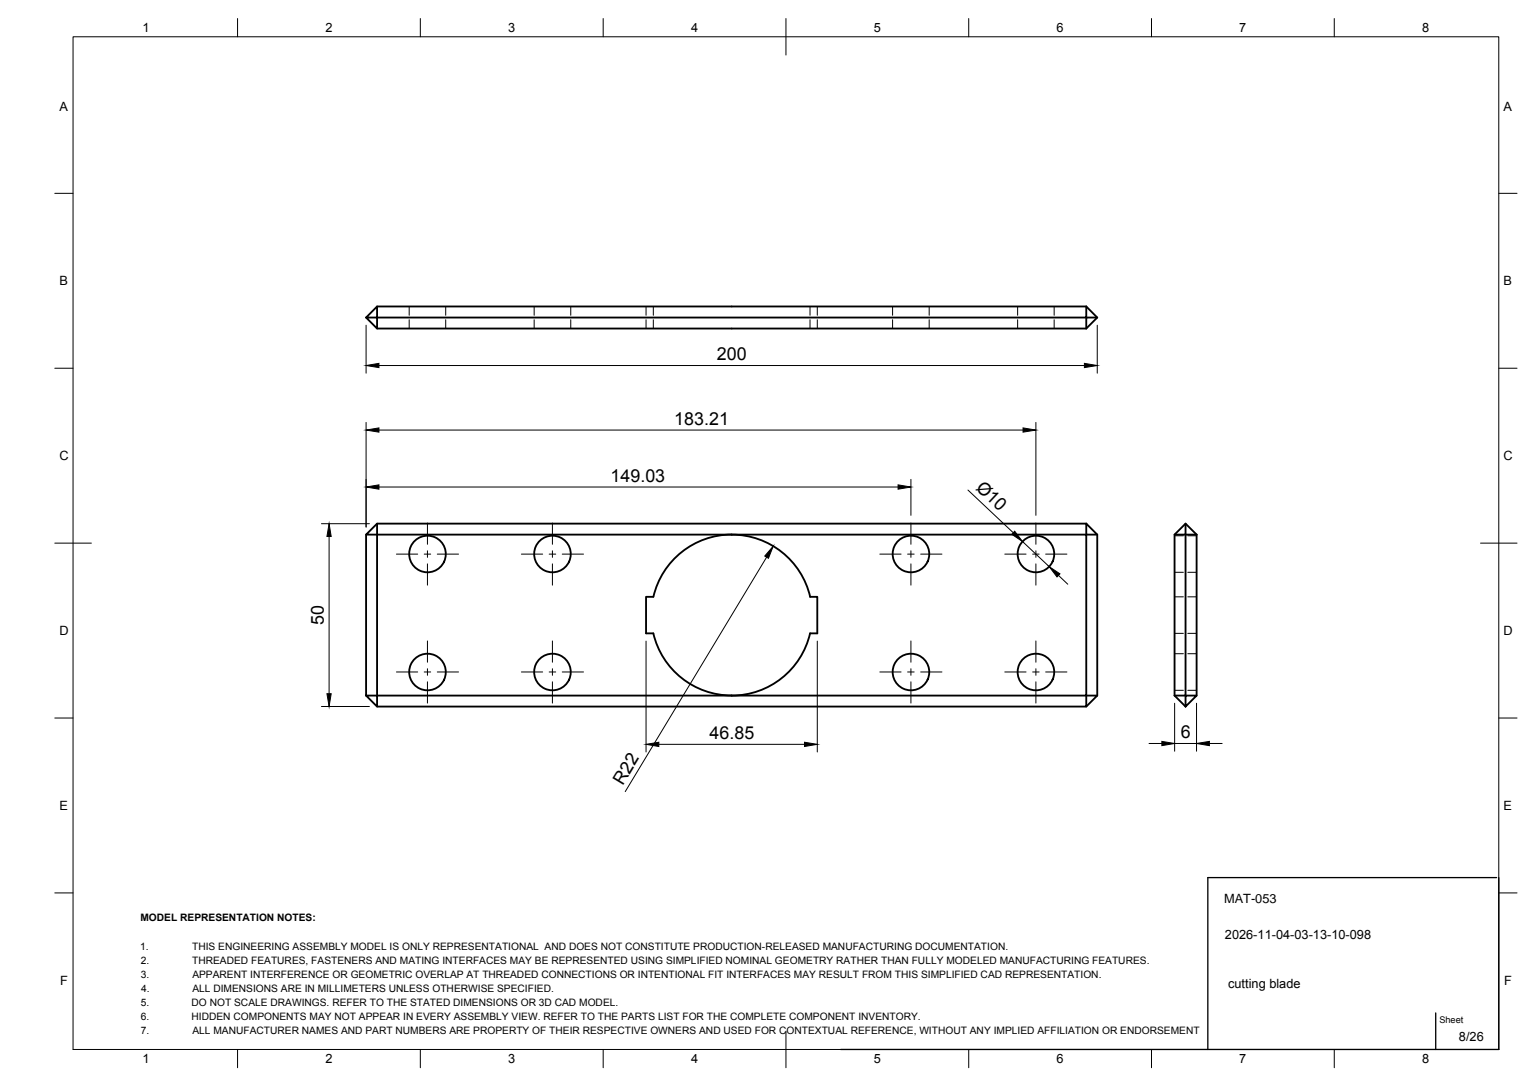
ISO-10303-21;
HEADER;
FILE_DESCRIPTION (('STEP AP214'),
    '1' );
FILE_NAME ('cutting blade.step',
    '2026-10-10T03:43:58',
    ( '' ),
    ( '' ),
    'SwSTEP 2.0',
    'SolidWorks 2026',
    '' );
FILE_SCHEMA (( 'AUTOMOTIVE_DESIGN' ));
ENDSEC;

DATA;
#169=CARTESIAN_POINT ( 'NONE',  ( 123.4242852856285566, 6.000000000000000000, 0.000000000000000000 ) ) ;
#175=PLANE ( 'NONE',  #51290 ) ;
#357=AXIS2_PLACEMENT_3D ( 'NONE', #51385, #66883, #65837 ) ;
#396=ORIENTED_EDGE ( 'NONE', *, *, #36645, .T. ) ;
#421=VECTOR ( 'NONE', #35144, 1000.000000000000000 ) ;
#435=APPLICATION_CONTEXT ( 'automotive_design' ) ;
#494=FACE_OUTER_BOUND ( 'NONE', #26933, .T. ) ;
#533=LINE ( 'NONE', #52947, #16766 ) ;
#715=CARTESIAN_POINT ( 'NONE',  ( 200.0000000000000000, 2.999999999999969802, -46.99999999999997158 ) ) ;
#779=CARTESIAN_POINT ( 'NONE',  ( 196.9999999999999716, 1.500000000000015321, -1.500000000000015321 ) ) ;
#839=DIRECTION ( 'NONE',  ( 0.7071067811865475727, 0.000000000000000000, -0.7071067811865475727 ) ) ;
#878=LINE ( 'NONE', #59590, #42830 ) ;
#897=CARTESIAN_POINT ( 'NONE',  ( 0.000000000000000000, 6.000000000000000000, -46.99999999999997158 ) ) ;
#978=DIRECTION ( 'NONE',  ( -0.000000000000000000, -1.000000000000000000, -0.000000000000000000 ) ) ;
#1008=LINE ( 'NONE', #43202, #21889 ) ;
#1056=CYLINDRICAL_SURFACE ( 'NONE', #3184, 5.000000000000018652 ) ;
#1109=CIRCLE ( 'NONE', #48227, 21.99999999999998579 ) ;
#1145=DIRECTION ( 'NONE',  ( -0.000000000000000000, -0.7071067811865474617, 0.7071067811865474617 ) ) ;
#1186=FACE_BOUND ( 'NONE', #2757, .T. ) ;
#1201=DIRECTION ( 'NONE',  ( -0.5773502691896255090, -0.5773502691896258421, 0.5773502691896258421 ) ) ;
#1207=ADVANCED_FACE ( 'NONE', ( #57854, #55337, #28257, #1186, #27560 ), #44439, .F. ) ;
#1231=LINE ( 'NONE', #29025, #57253 ) ;
#1239=DIRECTION ( 'NONE',  ( 0.7071067811865474617, -0.7071067811865474617, -0.000000000000000000 ) ) ;
#1254=VERTEX_POINT ( 'NONE', #27212 ) ;
#1260=EDGE_CURVE ( 'NONE', #42425, #65549, #28621, .T. ) ;
#1315=PLANE ( 'NONE',  #1532 ) ;
#1431=DIRECTION ( 'NONE',  ( 0.000000000000000000, 1.000000000000000000, 0.000000000000000000 ) ) ;
#1515=DIRECTION ( 'NONE',  ( 0.000000000000000000, 1.000000000000000000, -0.000000000000000000 ) ) ;
#1532=AXIS2_PLACEMENT_3D ( 'NONE', #12569, #6939, #17848 ) ;
#1616=ORIENTED_EDGE ( 'NONE', *, *, #7716, .T. ) ;
#1626=CARTESIAN_POINT ( 'NONE',  ( 16.78635691501517613, 6.000000000000000000, -4.435653166495499455 ) ) ;
#1709=CARTESIAN_POINT ( 'NONE',  ( 200.0000000000000000, 0.000000000000000000, -46.99999999999997158 ) ) ;
#1740=VECTOR ( 'NONE', #65545, 1000.000000000000000 ) ;
#1772=ORIENTED_EDGE ( 'NONE', *, *, #31156, .T. ) ;
#1902=DIRECTION ( 'NONE',  ( 0.000000000000000000, 0.000000000000000000, -1.000000000000000000 ) ) ;
#1942=CARTESIAN_POINT ( 'NONE',  ( 50.97490815085634352, 6.000000000000000000, -46.68900338898716029 ) ) ;
#1982=AXIS2_PLACEMENT_3D ( 'NONE', #37710, #69378, #69021 ) ;
#2065=CARTESIAN_POINT ( 'NONE',  ( 78.57571471437144339, 0.000000000000000000, -30.00000000000000355 ) ) ;
#2169=DIRECTION ( 'NONE',  ( -0.7071067811865474617, -0.000000000000000000, -0.7071067811865474617 ) ) ;
#2253=DIRECTION ( 'NONE',  ( 0.000000000000000000, 0.000000000000000000, -1.000000000000000000 ) ) ;
#2282=CARTESIAN_POINT ( 'NONE',  ( 183.2136430849847955, 6.000000000000000000, -41.68900338898720292 ) ) ;
#2313=CIRCLE ( 'NONE', #61839, 21.99999999999998579 ) ;
#2414=DIRECTION ( 'NONE',  ( 0.000000000000000000, 1.000000000000000000, -0.000000000000000000 ) ) ;
#2441=PLANE ( 'NONE',  #40587 ) ;
#2448=AXIS2_PLACEMENT_3D ( 'NONE', #61221, #56632, #34153 ) ;
#2451=DIRECTION ( 'NONE',  ( -0.000000000000000000, -1.000000000000000000, -0.000000000000000000 ) ) ;
#2481=EDGE_CURVE ( 'NONE', #65549, #11659, #47136, .T. ) ;
#2566=ORIENTED_EDGE ( 'NONE', *, *, #63693, .F. ) ;
#2616=DIRECTION ( 'NONE',  ( -0.7071067811865474617, 0.7071067811865474617, -0.000000000000000000 ) ) ;
#2621=ORIENTED_EDGE ( 'NONE', *, *, #25957, .T. ) ;
#2671=DIRECTION ( 'NONE',  ( -0.000000000000000000, -1.000000000000000000, -0.000000000000000000 ) ) ;
#2707=FACE_OUTER_BOUND ( 'NONE', #53949, .T. ) ;
#2757=EDGE_LOOP ( 'NONE', ( #15220, #28245 ) ) ;
#2839=CARTESIAN_POINT ( 'NONE',  ( 183.2136430849848239, 0.000000000000000000, -14.43565316649556074 ) ) ;
#3063=EDGE_LOOP ( 'NONE', ( #65576, #48668, #15693, #29611 ) ) ;
#3184=AXIS2_PLACEMENT_3D ( 'NONE', #43604, #65785, #22507 ) ;
#3357=ORIENTED_EDGE ( 'NONE', *, *, #27947, .T. ) ;
#3410=VECTOR ( 'NONE', #2671, 1000.000000000000000 ) ;
#3435=AXIS2_PLACEMENT_3D ( 'NONE', #57257, #35805, #24215 ) ;
#3493=EDGE_CURVE ( 'NONE', #67476, #41408, #39123, .T. ) ;
#3530=ORIENTED_EDGE ( 'NONE', *, *, #45276, .F. ) ;
#3676=LINE ( 'NONE', #56449, #63447 ) ;
#3686=DIRECTION ( 'NONE',  ( 0.000000000000000000, 0.000000000000000000, -1.000000000000000000 ) ) ;
#3694=ORIENTED_EDGE ( 'NONE', *, *, #20467, .T. ) ;
#3705=EDGE_LOOP ( 'NONE', ( #55339, #15386, #56019, #65378, #27658 ) ) ;
#3834=EDGE_CURVE ( 'NONE', #64271, #1254, #23024, .T. ) ;
#3913=VERTEX_POINT ( 'NONE', #61691 ) ;
#3955=DIRECTION ( 'NONE',  ( -0.000000000000000000, -1.000000000000000000, -0.000000000000000000 ) ) ;
#4029=CARTESIAN_POINT ( 'NONE',  ( 200.0000000000000000, 3.000000000000030198, -3.000000000000030198 ) ) ;
#4101=EDGE_LOOP ( 'NONE', ( #34045, #40743 ) ) ;
#4168=ORIENTED_EDGE ( 'NONE', *, *, #18126, .T. ) ;
#4278=ORIENTED_EDGE ( 'NONE', *, *, #64901, .F. ) ;
#4281=ORIENTED_EDGE ( 'NONE', *, *, #27062, .T. ) ;
#4315=CARTESIAN_POINT ( 'NONE',  ( 16.78635691501517613, 0.000000000000000000, -4.435653166495499455 ) ) ;
#4420=DIRECTION ( 'NONE',  ( 1.000000000000000000, -0.000000000000000000, -0.000000000000000000 ) ) ;
#4432=EDGE_CURVE ( 'NONE', #53754, #46832, #13689, .T. ) ;
#4537=DIRECTION ( 'NONE',  ( 0.000000000000000000, 1.000000000000000000, -0.000000000000000000 ) ) ;
#4544=CYLINDRICAL_SURFACE ( 'NONE', #15389, 5.000000000000000888 ) ;
#4601=ADVANCED_FACE ( 'NONE', ( #54409 ), #1315, .F. ) ;
#4627=AXIS2_PLACEMENT_3D ( 'NONE', #8850, #67257, #25026 ) ;
#4646=DIRECTION ( 'NONE',  ( 0.000000000000000000, 0.000000000000000000, 1.000000000000000000 ) ) ;
#4723=FACE_OUTER_BOUND ( 'NONE', #69286, .T. ) ;
#4726=ORIENTED_EDGE ( 'NONE', *, *, #60338, .T. ) ;
#4768=DIRECTION ( 'NONE',  ( 1.000000000000000000, 0.000000000000000000, 1.734723475976805517E-15 ) ) ;
#4785=EDGE_LOOP ( 'NONE', ( #23234, #53980 ) ) ;
#4794=DIRECTION ( 'NONE',  ( 0.000000000000000000, 0.000000000000000000, -1.000000000000000000 ) ) ;
#4937=CARTESIAN_POINT ( 'NONE',  ( 5.204170427930454100E-14, 6.000000000000000000, -30.00000000000021316 ) ) ;
#4941=AXIS2_PLACEMENT_3D ( 'NONE', #7124, #6773, #39149 ) ;
#4955=FACE_OUTER_BOUND ( 'NONE', #64021, .T. ) ;
#5076=EDGE_CURVE ( 'NONE', #50492, #67476, #66494, .T. ) ;
#5099=CARTESIAN_POINT ( 'NONE',  ( 149.0250918491436778, 0.000000000000000000, -4.435653166495538535 ) ) ;
#5123=AXIS2_PLACEMENT_3D ( 'NONE', #5757, #63827, #58199 ) ;
#5128=DIRECTION ( 'NONE',  ( -1.000000000000000000, 0.000000000000000000, 0.000000000000000000 ) ) ;
#5242=ORIENTED_EDGE ( 'NONE', *, *, #14158, .F. ) ;
#5316=LINE ( 'NONE', #10238, #50013 ) ;
#5338=CARTESIAN_POINT ( 'NONE',  ( 123.4242852856285566, 10.00000000000000000, -30.00000000000000000 ) ) ;
#5431=FACE_OUTER_BOUND ( 'NONE', #59546, .T. ) ;
#5461=EDGE_CURVE ( 'NONE', #17220, #64271, #10143, .T. ) ;
#5496=CARTESIAN_POINT ( 'NONE',  ( 76.57571471437145760, 0.000000000000000000, -30.00000000000000000 ) ) ;
#5497=FACE_BOUND ( 'NONE', #67109, .T. ) ;
#5558=ORIENTED_EDGE ( 'NONE', *, *, #20467, .F. ) ;
#5597=CIRCLE ( 'NONE', #40459, 5.000000000000018652 ) ;
#5637=ORIENTED_EDGE ( 'NONE', *, *, #14756, .T. ) ;
#5640=VERTEX_POINT ( 'NONE', #9729 ) ;
#5740=FACE_OUTER_BOUND ( 'NONE', #30395, .T. ) ;
#5757=CARTESIAN_POINT ( 'NONE',  ( 183.2136430849848239, 6.000000000000000000, -9.435653166495541200 ) ) ;
#5788=CIRCLE ( 'NONE', #2448, 4.999999999999990230 ) ;
#5944=VERTEX_POINT ( 'NONE', #17776 ) ;
#5971=VECTOR ( 'NONE', #26457, 1000.000000000000000 ) ;
#6015=AXIS2_PLACEMENT_3D ( 'NONE', #62685, #18728, #40188 ) ;
#6027=CYLINDRICAL_SURFACE ( 'NONE', #52139, 4.999999999999990230 ) ;
#6089=ORIENTED_EDGE ( 'NONE', *, *, #12217, .F. ) ;
#6097=DIRECTION ( 'NONE',  ( -0.000000000000000000, -0.7071067811865474617, -0.7071067811865474617 ) ) ;
#6148=VERTEX_POINT ( 'NONE', #9291 ) ;
#6166=EDGE_CURVE ( 'NONE', #44138, #3913, #52873, .T. ) ;
#6181=( GEOMETRIC_REPRESENTATION_CONTEXT ( 3 ) GLOBAL_UNCERTAINTY_ASSIGNED_CONTEXT ( ( #62024 ) ) GLOBAL_UNIT_ASSIGNED_CONTEXT ( ( #51907, #14959, #58221 ) ) REPRESENTATION_CONTEXT ( 'NONE', 'WORKASPACE' ) );
#6323=EDGE_CURVE ( 'NONE', #30445, #36476, #50644, .T. ) ;
#6355=CARTESIAN_POINT ( 'NONE',  ( 3.000000000000028866, 2.999999999999969802, 0.000000000000000000 ) ) ;
#6420=CARTESIAN_POINT ( 'NONE',  ( 196.9999999999999716, 2.999999999999969802, 0.000000000000000000 ) ) ;
#6461=EDGE_CURVE ( 'NONE', #60670, #23191, #10490, .T. ) ;
#6509=ORIENTED_EDGE ( 'NONE', *, *, #37316, .F. ) ;
#6538=ORIENTED_EDGE ( 'NONE', *, *, #17367, .T. ) ;
#6617=CARTESIAN_POINT ( 'NONE',  ( 50.97490815085634352, 6.000000000000000000, -41.68900338898716740 ) ) ;
#6648=EDGE_CURVE ( 'NONE', #36476, #52936, #41005, .T. ) ;
#6690=VERTEX_POINT ( 'NONE', #8674 ) ;
#6773=DIRECTION ( 'NONE',  ( -1.000000000000000000, 0.000000000000000000, 0.000000000000000000 ) ) ;
#6818=EDGE_LOOP ( 'NONE', ( #40697, #28804, #34762, #10078 ) ) ;
#6835=LINE ( 'NONE', #32189, #53156 ) ;
#6843=CIRCLE ( 'NONE', #67521, 4.999999999999990230 ) ;
#6939=DIRECTION ( 'NONE',  ( -1.734723475976805517E-15, 0.000000000000000000, -1.000000000000000000 ) ) ;
#6948=AXIS2_PLACEMENT_3D ( 'NONE', #19833, #41289, #36353 ) ;
#6972=CARTESIAN_POINT ( 'NONE',  ( 0.000000000000000000, 6.000000000000000000, -46.99999999999997158 ) ) ;
#6986=EDGE_CURVE ( 'NONE', #6690, #44138, #3676, .T. ) ;
#7064=LINE ( 'NONE', #33103, #61226 ) ;
#7089=VERTEX_POINT ( 'NONE', #32140 ) ;
#7104=DIRECTION ( 'NONE',  ( 0.000000000000000000, 0.000000000000000000, 1.000000000000000000 ) ) ;
#7108=CIRCLE ( 'NONE', #14983, 5.000000000000018652 ) ;
#7124=CARTESIAN_POINT ( 'NONE',  ( 123.4242852856285566, 10.00000000000000000, -20.00000000000000000 ) ) ;
#7145=ORIENTED_EDGE ( 'NONE', *, *, #29514, .T. ) ;
#7165=EDGE_CURVE ( 'NONE', #45847, #62711, #39167, .T. ) ;
#7169=VECTOR ( 'NONE', #47823, 1000.000000000000114 ) ;
#7198=CARTESIAN_POINT ( 'NONE',  ( 198.4999999999999716, 4.499999999999984901, -3.000000000000030198 ) ) ;
#7220=VECTOR ( 'NONE', #55627, 1000.000000000000114 ) ;
#7324=EDGE_CURVE ( 'NONE', #42425, #30796, #49253, .T. ) ;
#7466=CARTESIAN_POINT ( 'NONE',  ( 149.0250918491436494, 6.000000000000000000, -36.68900338898720292 ) ) ;
#7473=CIRCLE ( 'NONE', #20911, 4.999999999999990230 ) ;
#7553=LINE ( 'NONE', #44477, #68985 ) ;
#7574=ORIENTED_EDGE ( 'NONE', *, *, #3834, .F. ) ;
#7587=CARTESIAN_POINT ( 'NONE',  ( 196.9999999999999716, 4.499999999999984901, -48.49999999999998579 ) ) ;
#7647=DIRECTION ( 'NONE',  ( 0.000000000000000000, 0.000000000000000000, -1.000000000000000000 ) ) ;
#7685=ORIENTED_EDGE ( 'NONE', *, *, #32000, .T. ) ;
#7701=DIRECTION ( 'NONE',  ( 0.000000000000000000, 1.000000000000000000, 0.000000000000000000 ) ) ;
#7716=EDGE_CURVE ( 'NONE', #10774, #9838, #42015, .T. ) ;
#7755=VECTOR ( 'NONE', #58395, 1000.000000000000000 ) ;
#7779=EDGE_CURVE ( 'NONE', #44138, #63882, #58869, .T. ) ;
#8093=EDGE_CURVE ( 'NONE', #30336, #59608, #10600, .T. ) ;
#8143=ORIENTED_EDGE ( 'NONE', *, *, #37114, .F. ) ;
#8183=CARTESIAN_POINT ( 'NONE',  ( 3.000000000000028866, 3.000000000000030198, 0.000000000000000000 ) ) ;
#8253=( GEOMETRIC_REPRESENTATION_CONTEXT ( 3 ) GLOBAL_UNCERTAINTY_ASSIGNED_CONTEXT ( ( #56404 ) ) GLOBAL_UNIT_ASSIGNED_CONTEXT ( ( #66641, #61689, #39207 ) ) REPRESENTATION_CONTEXT ( 'NONE', 'WORKASPACE' ) );
#8319=DIRECTION ( 'NONE',  ( 1.000000000000000000, 0.000000000000000000, 0.000000000000000000 ) ) ;
#8373=DIRECTION ( 'NONE',  ( 0.000000000000000000, 0.000000000000000000, -1.000000000000000000 ) ) ;
#8472=FACE_OUTER_BOUND ( 'NONE', #38130, .T. ) ;
#8514=VECTOR ( 'NONE', #4420, 1000.000000000000000 ) ;
#8518=AXIS2_PLACEMENT_3D ( 'NONE', #27196, #47274, #47958 ) ;
#8530=EDGE_CURVE ( 'NONE', #53590, #18148, #7473, .T. ) ;
#8544=PLANE ( 'NONE',  #22300 ) ;
#8547=LINE ( 'NONE', #58106, #60205 ) ;
#8625=ORIENTED_EDGE ( 'NONE', *, *, #32000, .F. ) ;
#8629=DIRECTION ( 'NONE',  ( 0.000000000000000000, -0.7071067811865474617, 0.7071067811865474617 ) ) ;
#8637=DIRECTION ( 'NONE',  ( 0.000000000000000000, -1.000000000000000000, 0.000000000000000000 ) ) ;
#8674=CARTESIAN_POINT ( 'NONE',  ( 3.000000000000028866, 6.000000000000000000, -3.000000000000030198 ) ) ;
#8754=DIRECTION ( 'NONE',  ( -0.000000000000000000, -1.000000000000000000, -0.000000000000000000 ) ) ;
#8806=DIRECTION ( 'NONE',  ( 0.000000000000000000, 0.000000000000000000, -1.000000000000000000 ) ) ;
#8824=DIRECTION ( 'NONE',  ( 0.000000000000000000, 1.000000000000000000, 0.000000000000000000 ) ) ;
#8850=CARTESIAN_POINT ( 'NONE',  ( -2.775557561562891351E-14, 3.000000000000030198, -50.00000000000000000 ) ) ;
#8855=ORIENTED_EDGE ( 'NONE', *, *, #12862, .F. ) ;
#8968=VERTEX_POINT ( 'NONE', #60893 ) ;
#9045=EDGE_LOOP ( 'NONE', ( #5242, #53942, #39507, #50271 ) ) ;
#9066=CARTESIAN_POINT ( 'NONE',  ( 121.4242852856285566, 6.000000000000000000, -20.00000000000000000 ) ) ;
#9085=DIRECTION ( 'NONE',  ( 0.000000000000000000, 0.000000000000000000, -1.000000000000000000 ) ) ;
#9124=AXIS2_PLACEMENT_3D ( 'NONE', #12076, #1515, #28240 ) ;
#9125=AXIS2_PLACEMENT_3D ( 'NONE', #27577, #1201, #49369 ) ;
#9291=CARTESIAN_POINT ( 'NONE',  ( 78.57571471437145760, 0.000000000000000000, -20.00000000000000000 ) ) ;
#9319=DIRECTION ( 'NONE',  ( -0.5773502691896258421, -0.5773502691896258421, -0.5773502691896258421 ) ) ;
#9380=ADVANCED_FACE ( 'NONE', ( #36213 ), #31622, .F. ) ;
#9400=ORIENTED_EDGE ( 'NONE', *, *, #44188, .T. ) ;
#9421=ORIENTED_EDGE ( 'NONE', *, *, #64314, .T. ) ;
#9457=ADVANCED_FACE ( 'NONE', ( #20369 ), #4544, .F. ) ;
#9513=CIRCLE ( 'NONE', #54419, 21.99999999999998579 ) ;
#9591=EDGE_LOOP ( 'NONE', ( #62598, #61913, #37505, #11408, #50798, #48930, #15590, #30937 ) ) ;
#9674=VECTOR ( 'NONE', #6097, 1000.000000000000114 ) ;
#9729=CARTESIAN_POINT ( 'NONE',  ( -2.609024107869115977E-14, 3.000000000000030198, -46.99999999999997158 ) ) ;
#9838=VERTEX_POINT ( 'NONE', #32576 ) ;
#9897=CYLINDRICAL_SURFACE ( 'NONE', #31651, 21.99999999999998579 ) ;
#10012=DIRECTION ( 'NONE',  ( 1.000000000000000000, 0.000000000000000000, 0.000000000000000000 ) ) ;
#10024=PLANE ( 'NONE',  #29251 ) ;
#10078=ORIENTED_EDGE ( 'NONE', *, *, #33445, .F. ) ;
#10104=DIRECTION ( 'NONE',  ( 0.000000000000000000, 0.000000000000000000, -1.000000000000000000 ) ) ;
#10143=LINE ( 'NONE', #59362, #36435 ) ;
#10216=DIRECTION ( 'NONE',  ( -0.7071067811865474617, 0.7071067811865474617, 0.000000000000000000 ) ) ;
#10224=CARTESIAN_POINT ( 'NONE',  ( 99.99999999999997158, 6.000000000000000000, -25.00000000000000000 ) ) ;
#10238=CARTESIAN_POINT ( 'NONE',  ( 16.78635691501517613, 6.000000000000000000, -36.68900338898716740 ) ) ;
#10314=ORIENTED_EDGE ( 'NONE', *, *, #42088, .F. ) ;
#10378=PRODUCT_CONTEXT ( 'NONE', #41742, 'mechanical' ) ;
#10389=EDGE_CURVE ( 'NONE', #41408, #31811, #31037, .T. ) ;
#10396=CIRCLE ( 'NONE', #36269, 4.999999999999996447 ) ;
#10399=PLANE ( 'NONE',  #11397 ) ;
#10422=PLANE ( 'NONE',  #35855 ) ;
#10452=ORIENTED_EDGE ( 'NONE', *, *, #18428, .F. ) ;
#10477=LINE ( 'NONE', #47764, #48342 ) ;
#10488=VERTEX_POINT ( 'NONE', #26095 ) ;
#10490=LINE ( 'NONE', #47427, #26395 ) ;
#10542=ADVANCED_FACE ( 'NONE', ( #51456 ), #40889, .F. ) ;
#10543=EDGE_LOOP ( 'NONE', ( #41686, #46294, #63996, #41184, #25059 ) ) ;
#10600=LINE ( 'NONE', #5338, #11868 ) ;
#10607=DIRECTION ( 'NONE',  ( 0.7071067811865475727, -0.7071067811865475727, 0.000000000000000000 ) ) ;
#10749=CIRCLE ( 'NONE', #52337, 4.999999999999997335 ) ;
#10774=VERTEX_POINT ( 'NONE', #9066 ) ;
#10905=EDGE_LOOP ( 'NONE', ( #65462, #4726, #57157, #8855 ) ) ;
#10968=CARTESIAN_POINT ( 'NONE',  ( 196.9999999999999716, 1.500000000000015321, -48.49999999999998579 ) ) ;
#11042=DIRECTION ( 'NONE',  ( -0.000000000000000000, -1.000000000000000000, -0.000000000000000000 ) ) ;
#11068=ORIENTED_EDGE ( 'NONE', *, *, #54016, .F. ) ;
#11085=PLANE ( 'NONE',  #16711 ) ;
#11100=CARTESIAN_POINT ( 'NONE',  ( 50.97490815085634352, 6.000000000000000000, -9.435653166495500344 ) ) ;
#11157=VECTOR ( 'NONE', #55500, 1000.000000000000000 ) ;
#11216=DIRECTION ( 'NONE',  ( 0.000000000000000000, -0.7071067811865475727, 0.7071067811865475727 ) ) ;
#11232=ORIENTED_EDGE ( 'NONE', *, *, #23537, .F. ) ;
#11246=DIRECTION ( 'NONE',  ( 0.000000000000000000, 1.000000000000000000, 0.000000000000000000 ) ) ;
#11328=ADVANCED_FACE ( 'NONE', ( #494 ), #64865, .F. ) ;
#11329=ORIENTED_EDGE ( 'NONE', *, *, #32716, .T. ) ;
#11389=CARTESIAN_POINT ( 'NONE',  ( 0.000000000000000000, 6.000000000000000000, -3.000000000000030198 ) ) ;
#11397=AXIS2_PLACEMENT_3D ( 'NONE', #37835, #5128, #64569 ) ;
#11408=ORIENTED_EDGE ( 'NONE', *, *, #24486, .F. ) ;
#11474=CARTESIAN_POINT ( 'NONE',  ( 76.57571471437145760, 6.000000000000000000, -30.00000000000000000 ) ) ;
#11505=CARTESIAN_POINT ( 'NONE',  ( 183.2136430849848239, 6.000000000000000000, -14.43565316649556074 ) ) ;
#11533=ORIENTED_EDGE ( 'NONE', *, *, #57029, .T. ) ;
#11559=DIRECTION ( 'NONE',  ( 0.000000000000000000, 0.000000000000000000, 1.000000000000000000 ) ) ;
#11586=ORIENTED_EDGE ( 'NONE', *, *, #14158, .T. ) ;
#11618=LINE ( 'NONE', #55582, #66913 ) ;
#11619=FACE_OUTER_BOUND ( 'NONE', #21673, .T. ) ;
#11659=VERTEX_POINT ( 'NONE', #39437 ) ;
#11741=ORIENTED_EDGE ( 'NONE', *, *, #14944, .T. ) ;
#11795=AXIS2_PLACEMENT_3D ( 'NONE', #35959, #31375, #58102 ) ;
#11800=AXIS2_PLACEMENT_3D ( 'NONE', #43232, #65057, #64706 ) ;
#11862=VECTOR ( 'NONE', #57382, 1000.000000000000000 ) ;
#11868=VECTOR ( 'NONE', #16576, 1000.000000000000000 ) ;
#11893=CARTESIAN_POINT ( 'NONE',  ( 183.2136430849847955, 6.000000000000000000, -36.68900338898718871 ) ) ;
#11987=ADVANCED_FACE ( 'NONE', ( #16503 ), #26380, .T. ) ;
#12076=CARTESIAN_POINT ( 'NONE',  ( 149.0250918491436778, 6.000000000000000000, -9.435653166495526989 ) ) ;
#12098=CARTESIAN_POINT ( 'NONE',  ( 50.97490815085634352, 6.000000000000000000, -41.68900338898716740 ) ) ;
#12136=VERTEX_POINT ( 'NONE', #29490 ) ;
#12152=FACE_OUTER_BOUND ( 'NONE', #3705, .T. ) ;
#12165=ORIENTED_EDGE ( 'NONE', *, *, #42088, .T. ) ;
#12194=DIRECTION ( 'NONE',  ( 0.000000000000000000, 0.000000000000000000, 1.000000000000000000 ) ) ;
#12214=FACE_OUTER_BOUND ( 'NONE', #69097, .T. ) ;
#12217=EDGE_CURVE ( 'NONE', #22100, #56047, #13186, .T. ) ;
#12223=ADVANCED_FACE ( 'NONE', ( #67155 ), #52333, .F. ) ;
#12280=ORIENTED_EDGE ( 'NONE', *, *, #25736, .F. ) ;
#12287=ORIENTED_EDGE ( 'NONE', *, *, #27947, .F. ) ;
#12321=CARTESIAN_POINT ( 'NONE',  ( 16.78635691501517613, 6.000000000000000000, -46.68900338898716029 ) ) ;
#12420=DIRECTION ( 'NONE',  ( 0.000000000000000000, 0.000000000000000000, 1.000000000000000000 ) ) ;
#12569=CARTESIAN_POINT ( 'NONE',  ( 76.57571471437145760, 10.00000000000000000, -30.00000000000000000 ) ) ;
#12605=EDGE_LOOP ( 'NONE', ( #13770, #54497 ) ) ;
#12656=LINE ( 'NONE', #13015, #66385 ) ;
#12658=DIRECTION ( 'NONE',  ( 0.000000000000000000, 0.000000000000000000, 1.000000000000000000 ) ) ;
#12754=ORIENTED_EDGE ( 'NONE', *, *, #12217, .T. ) ;
#12785=EDGE_CURVE ( 'NONE', #68142, #60670, #36778, .T. ) ;
#12820=ORIENTED_EDGE ( 'NONE', *, *, #31011, .T. ) ;
#12827=DIRECTION ( 'NONE',  ( 0.000000000000000000, 0.000000000000000000, -1.000000000000000000 ) ) ;
#12862=EDGE_CURVE ( 'NONE', #52936, #36476, #16571, .T. ) ;
#12875=EDGE_CURVE ( 'NONE', #65549, #44262, #29212, .T. ) ;
#12940=EDGE_LOOP ( 'NONE', ( #6089, #37237 ) ) ;
#12965=ORIENTED_EDGE ( 'NONE', *, *, #14226, .T. ) ;
#12973=ORIENTED_EDGE ( 'NONE', *, *, #3493, .T. ) ;
#13011=DIRECTION ( 'NONE',  ( 1.000000000000000000, 0.000000000000000000, 0.000000000000000000 ) ) ;
#13015=CARTESIAN_POINT ( 'NONE',  ( 3.000000000000028866, 0.000000000000000000, -3.000000000000030198 ) ) ;
#13186=CIRCLE ( 'NONE', #15380, 5.000000000000018652 ) ;
#13301=ADVANCED_FACE ( 'NONE', ( #58606, #58956, #5497, #54005, #27291 ), #10422, .F. ) ;
#13407=DIRECTION ( 'NONE',  ( 0.7071067811865474617, -0.000000000000000000, -0.7071067811865474617 ) ) ;
#13601=CYLINDRICAL_SURFACE ( 'NONE', #15479, 4.999999999999997335 ) ;
#13624=DIRECTION ( 'NONE',  ( -1.000000000000000000, 0.000000000000000000, 0.000000000000000000 ) ) ;
#13689=LINE ( 'NONE', #29515, #421 ) ;
#13770=ORIENTED_EDGE ( 'NONE', *, *, #31594, .T. ) ;
#13810=DIRECTION ( 'NONE',  ( 0.000000000000000000, -1.000000000000000000, 0.000000000000000000 ) ) ;
#13866=MECHANICAL_DESIGN_GEOMETRIC_PRESENTATION_REPRESENTATION('',(#34118),#8253);
#13882=ORIENTED_EDGE ( 'NONE', *, *, #57267, .T. ) ;
#13947=DIRECTION ( 'NONE',  ( -0.000000000000000000, -1.000000000000000000, -0.000000000000000000 ) ) ;
#13985=LINE ( 'NONE', #35443, #67376 ) ;
#14020=EDGE_LOOP ( 'NONE', ( #44092, #12820, #26767, #29878 ) ) ;
#14048=ORIENTED_EDGE ( 'NONE', *, *, #50300, .F. ) ;
#14158=EDGE_CURVE ( 'NONE', #68142, #39369, #28716, .T. ) ;
#14226=EDGE_CURVE ( 'NONE', #6690, #3913, #50854, .T. ) ;
#14305=DIRECTION ( 'NONE',  ( 0.000000000000000000, 1.000000000000000000, 0.000000000000000000 ) ) ;
#14313=DIRECTION ( 'NONE',  ( 0.000000000000000000, 1.000000000000000000, 0.000000000000000000 ) ) ;
#14350=FACE_OUTER_BOUND ( 'NONE', #10905, .T. ) ;
#14410=LINE ( 'NONE', #19329, #47763 ) ;
#14482=ORIENTED_EDGE ( 'NONE', *, *, #68300, .F. ) ;
#14571=CARTESIAN_POINT ( 'NONE',  ( 1.500000000000013545, 3.000000000000030198, -1.500000000000014211 ) ) ;
#14609=EDGE_CURVE ( 'NONE', #41760, #32688, #5597, .T. ) ;
#14756=EDGE_CURVE ( 'NONE', #22171, #66403, #33784, .T. ) ;
#14762=EDGE_LOOP ( 'NONE', ( #54071, #67113, #43671, #2566 ) ) ;
#14777=EDGE_CURVE ( 'NONE', #63181, #41760, #33036, .T. ) ;
#14855=PLANE ( 'NONE',  #29532 ) ;
#14887=CYLINDRICAL_SURFACE ( 'NONE', #6948, 4.999999999999997335 ) ;
#14889=DIRECTION ( 'NONE',  ( 0.000000000000000000, 0.000000000000000000, 1.000000000000000000 ) ) ;
#14944=EDGE_CURVE ( 'NONE', #31811, #12136, #2313, .T. ) ;
#14946=CARTESIAN_POINT ( 'NONE',  ( 0.000000000000000000, 0.000000000000000000, 0.000000000000000000 ) ) ;
#14959=( NAMED_UNIT ( * ) PLANE_ANGLE_UNIT ( ) SI_UNIT ( $, .RADIAN. ) );
#14983=AXIS2_PLACEMENT_3D ( 'NONE', #49648, #53877, #21533 ) ;
#15193=CYLINDRICAL_SURFACE ( 'NONE', #11795, 4.999999999999997335 ) ;
#15220=ORIENTED_EDGE ( 'NONE', *, *, #25957, .F. ) ;
#15281=AXIS2_PLACEMENT_3D ( 'NONE', #68874, #16109, #20351 ) ;
#15289=CARTESIAN_POINT ( 'NONE',  ( 0.000000000000000000, 6.000000000000000000, -20.00000000000000000 ) ) ;
#15326=VECTOR ( 'NONE', #66032, 1000.000000000000000 ) ;
#15380=AXIS2_PLACEMENT_3D ( 'NONE', #56932, #35116, #46017 ) ;
#15386=ORIENTED_EDGE ( 'NONE', *, *, #12875, .F. ) ;
#15389=AXIS2_PLACEMENT_3D ( 'NONE', #53397, #47786, #69248 ) ;
#15479=AXIS2_PLACEMENT_3D ( 'NONE', #23477, #13947, #7647 ) ;
#15557=ORIENTED_EDGE ( 'NONE', *, *, #67271, .F. ) ;
#15590=ORIENTED_EDGE ( 'NONE', *, *, #35893, .T. ) ;
#15693=ORIENTED_EDGE ( 'NONE', *, *, #31734, .F. ) ;
#16099=DIRECTION ( 'NONE',  ( 0.000000000000000000, 1.000000000000000000, 0.000000000000000000 ) ) ;
#16109=DIRECTION ( 'NONE',  ( 0.000000000000000000, 1.000000000000000000, 0.000000000000000000 ) ) ;
#16191=LINE ( 'NONE', #715, #56817 ) ;
#16256=CARTESIAN_POINT ( 'NONE',  ( 149.0250918491436494, 0.000000000000000000, -36.68900338898720292 ) ) ;
#16350=CARTESIAN_POINT ( 'NONE',  ( 16.78635691501517613, 6.000000000000000000, -41.68900338898716740 ) ) ;
#16424=DIRECTION ( 'NONE',  ( -0.000000000000000000, -1.000000000000000000, -0.000000000000000000 ) ) ;
#16503=FACE_OUTER_BOUND ( 'NONE', #41391, .T. ) ;
#16571=CIRCLE ( 'NONE', #59247, 4.999999999999997335 ) ;
#16576=DIRECTION ( 'NONE',  ( -0.000000000000000000, -1.000000000000000000, -0.000000000000000000 ) ) ;
#16605=DIRECTION ( 'NONE',  ( 0.000000000000000000, 1.000000000000000000, 0.000000000000000000 ) ) ;
#16662=CARTESIAN_POINT ( 'NONE',  ( 0.000000000000000000, 6.000000000000000000, 0.000000000000000000 ) ) ;
#16711=AXIS2_PLACEMENT_3D ( 'NONE', #23409, #55038, #27259 ) ;
#16731=PLANE ( 'NONE',  #65801 ) ;
#16766=VECTOR ( 'NONE', #53972, 1000.000000000000000 ) ;
#16842=CARTESIAN_POINT ( 'NONE',  ( 0.000000000000000000, 3.000000000000030198, 0.000000000000000000 ) ) ;
#16845=CARTESIAN_POINT ( 'NONE',  ( 183.2136430849847955, 6.000000000000000000, -46.68900338898722424 ) ) ;
#16874=ORIENTED_EDGE ( 'NONE', *, *, #10389, .F. ) ;
#16903=CARTESIAN_POINT ( 'NONE',  ( 78.57571471437145760, 6.000000000000000000, -20.00000000000000000 ) ) ;
#17008=DIRECTION ( 'NONE',  ( 0.000000000000000000, 1.000000000000000000, -0.000000000000000000 ) ) ;
#17151=ADVANCED_FACE ( 'NONE', ( #46707 ), #19279, .F. ) ;
#17183=DIRECTION ( 'NONE',  ( -0.7071067811865474617, -0.7071067811865474617, 1.196099074440432629E-16 ) ) ;
#17220=VERTEX_POINT ( 'NONE', #17370 ) ;
#17283=ORIENTED_EDGE ( 'NONE', *, *, #36081, .F. ) ;
#17367=EDGE_CURVE ( 'NONE', #6690, #17220, #55711, .T. ) ;
#17370=CARTESIAN_POINT ( 'NONE',  ( 99.99999999999997158, 6.000000000000000000, -3.000000000000030198 ) ) ;
#17375=ADVANCED_FACE ( 'NONE', ( #54294 ), #17740, .T. ) ;
#17387=DIRECTION ( 'NONE',  ( 0.000000000000000000, 0.000000000000000000, -1.000000000000000000 ) ) ;
#17406=ORIENTED_EDGE ( 'NONE', *, *, #45812, .T. ) ;
#17431=CIRCLE ( 'NONE', #32011, 5.000000000000018652 ) ;
#17482=ORIENTED_EDGE ( 'NONE', *, *, #6648, .T. ) ;
#17550=CARTESIAN_POINT ( 'NONE',  ( 50.97490815085634352, 0.000000000000000000, -36.68900338898716740 ) ) ;
#17578=PRODUCT_DEFINITION_SHAPE ( 'NONE', 'NONE',  #38320 ) ;
#17584=EDGE_LOOP ( 'NONE', ( #46465, #58255, #4281, #68143 ) ) ;
#17642=CARTESIAN_POINT ( 'NONE',  ( -2.609024107869115977E-14, 3.000000000000030198, -46.99999999999997158 ) ) ;
#17662=CARTESIAN_POINT ( 'NONE',  ( 3.000000000000004441, 2.999999999999969802, -50.00000000000000000 ) ) ;
#17740=PLANE ( 'NONE',  #9125 ) ;
#17772=FACE_OUTER_BOUND ( 'NONE', #51618, .T. ) ;
#17776=CARTESIAN_POINT ( 'NONE',  ( 50.97490815085634352, 6.000000000000000000, -4.435653166495503896 ) ) ;
#17825=CARTESIAN_POINT ( 'NONE',  ( 0.000000000000000000, 0.000000000000000000, -3.000000000000030198 ) ) ;
#17848=DIRECTION ( 'NONE',  ( -1.000000000000000000, 0.000000000000000000, 1.734723475976805517E-15 ) ) ;
#18098=DIRECTION ( 'NONE',  ( 0.000000000000000000, 1.000000000000000000, -0.000000000000000000 ) ) ;
#18126=EDGE_CURVE ( 'NONE', #3913, #63882, #12656, .T. ) ;
#18148=VERTEX_POINT ( 'NONE', #18625 ) ;
#18219=CARTESIAN_POINT ( 'NONE',  ( 3.000000000000004441, 0.000000000000000000, -46.99999999999997158 ) ) ;
#18349=DIRECTION ( 'NONE',  ( -0.5773502691896258421, 0.5773502691896257311, -0.5773502691896257311 ) ) ;
#18428=EDGE_CURVE ( 'NONE', #51453, #6148, #10477, .T. ) ;
#18476=CARTESIAN_POINT ( 'NONE',  ( 78.57571471437145760, 6.000000000000000000, -30.00000000000000000 ) ) ;
#18503=AXIS2_PLACEMENT_3D ( 'NONE', #57279, #8754, #41447 ) ;
#18506=ORIENTED_EDGE ( 'NONE', *, *, #27230, .T. ) ;
#18625=CARTESIAN_POINT ( 'NONE',  ( 149.0250918491436778, 0.000000000000000000, -14.43565316649551811 ) ) ;
#18642=ORIENTED_EDGE ( 'NONE', *, *, #6323, .F. ) ;
#18728=DIRECTION ( 'NONE',  ( 0.000000000000000000, 1.000000000000000000, 0.000000000000000000 ) ) ;
#18785=SURFACE_STYLE_USAGE ( .BOTH. , #28648 ) ;
#18794=DIRECTION ( 'NONE',  ( -0.000000000000000000, -1.000000000000000000, -0.000000000000000000 ) ) ;
#18853=DIRECTION ( 'NONE',  ( -0.7071067811865474617, -0.7071067811865474617, 3.951729029292866070E-16 ) ) ;
#19150=CARTESIAN_POINT ( 'NONE',  ( 3.000000000000030198, 6.000000000000000000, -1.665334536937751377E-15 ) ) ;
#19176=EDGE_LOOP ( 'NONE', ( #52915, #67730, #44469, #49002, #51732 ) ) ;
#19224=ADVANCED_FACE ( 'NONE', ( #4955 ), #9897, .F. ) ;
#19279=CYLINDRICAL_SURFACE ( 'NONE', #37220, 4.999999999999990230 ) ;
#19329=CARTESIAN_POINT ( 'NONE',  ( 149.0250918491436778, 6.000000000000000000, -4.435653166495538535 ) ) ;
#19385=ORIENTED_EDGE ( 'NONE', *, *, #8093, .T. ) ;
#19427=FACE_OUTER_BOUND ( 'NONE', #3063, .T. ) ;
#19455=AXIS2_PLACEMENT_3D ( 'NONE', #60770, #34051, #24201 ) ;
#19504=CIRCLE ( 'NONE', #25149, 21.99999999999998579 ) ;
#19545=ADVANCED_FACE ( 'NONE', ( #68795 ), #10399, .F. ) ;
#19617=CYLINDRICAL_SURFACE ( 'NONE', #3435, 4.999999999999997335 ) ;
#19751=ORIENTED_EDGE ( 'NONE', *, *, #54869, .F. ) ;
#19833=CARTESIAN_POINT ( 'NONE',  ( 16.78635691501517613, 6.000000000000000000, -41.68900338898716740 ) ) ;
#19843=VECTOR ( 'NONE', #23519, 1000.000000000000000 ) ;
#20040=AXIS2_PLACEMENT_3D ( 'NONE', #43514, #16099, #58653 ) ;
#20230=ORIENTED_EDGE ( 'NONE', *, *, #51610, .F. ) ;
#20249=LINE ( 'NONE', #25548, #8514 ) ;
#20319=DIRECTION ( 'NONE',  ( -0.000000000000000000, -1.000000000000000000, -0.000000000000000000 ) ) ;
#20324=CARTESIAN_POINT ( 'NONE',  ( 149.0250918491436494, 0.000000000000000000, -46.68900338898718161 ) ) ;
#20351=DIRECTION ( 'NONE',  ( 0.000000000000000000, 0.000000000000000000, 1.000000000000000000 ) ) ;
#20369=FACE_OUTER_BOUND ( 'NONE', #35571, .T. ) ;
#20467=EDGE_CURVE ( 'NONE', #50282, #53754, #59748, .T. ) ;
#20506=CARTESIAN_POINT ( 'NONE',  ( 16.78635691501517613, 6.000000000000000000, -14.43565316649550034 ) ) ;
#20517=EDGE_LOOP ( 'NONE', ( #12973, #57054, #56981 ) ) ;
#20518=ORIENTED_EDGE ( 'NONE', *, *, #14609, .F. ) ;
#20524=DIRECTION ( 'NONE',  ( -0.7071067811865477948, 2.775557561562891967E-17, -0.7071067811865473507 ) ) ;
#20526=DIRECTION ( 'NONE',  ( 0.7071067811865474617, 0.7071067811865474617, 0.000000000000000000 ) ) ;
#20564=FACE_BOUND ( 'NONE', #34264, .T. ) ;
#20670=FACE_OUTER_BOUND ( 'NONE', #6818, .T. ) ;
#20803=VECTOR ( 'NONE', #54886, 1000.000000000000000 ) ;
#20911=AXIS2_PLACEMENT_3D ( 'NONE', #50593, #2414, #10104 ) ;
#21155=ORIENTED_EDGE ( 'NONE', *, *, #2481, .F. ) ;
#21215=CARTESIAN_POINT ( 'NONE',  ( 99.99999999999997158, 6.000000000000000000, -25.00000000000000000 ) ) ;
#21396=ORIENTED_EDGE ( 'NONE', *, *, #56242, .F. ) ;
#21456=LINE ( 'NONE', #4937, #56600 ) ;
#21458=CIRCLE ( 'NONE', #43888, 4.999999999999990230 ) ;
#21533=DIRECTION ( 'NONE',  ( 0.000000000000000000, 0.000000000000000000, -1.000000000000000000 ) ) ;
#21584=CARTESIAN_POINT ( 'NONE',  ( 3.000000000000028866, 0.000000000000000000, -3.000000000000030198 ) ) ;
#21601=FACE_BOUND ( 'NONE', #12605, .T. ) ;
#21673=EDGE_LOOP ( 'NONE', ( #12965, #26989, #61676 ) ) ;
#21693=FACE_OUTER_BOUND ( 'NONE', #66089, .T. ) ;
#21697=VERTEX_POINT ( 'NONE', #25175 ) ;
#21889=VECTOR ( 'NONE', #22460, 1000.000000000000000 ) ;
#21935=PLANE ( 'NONE',  #43210 ) ;
#21938=DIRECTION ( 'NONE',  ( -0.000000000000000000, 0.7071067811865474617, -0.7071067811865474617 ) ) ;
#21948=DIRECTION ( 'NONE',  ( -1.000000000000000000, 0.000000000000000000, 0.000000000000000000 ) ) ;
#21954=VECTOR ( 'NONE', #13624, 1000.000000000000000 ) ;
#21956=VECTOR ( 'NONE', #22623, 1000.000000000000000 ) ;
#21996=VECTOR ( 'NONE', #17183, 1000.000000000000114 ) ;
#21999=EDGE_CURVE ( 'NONE', #50676, #46832, #34127, .T. ) ;
#22100=VERTEX_POINT ( 'NONE', #57951 ) ;
#22103=CARTESIAN_POINT ( 'NONE',  ( 50.97490815085634352, 0.000000000000000000, -4.435653166495503896 ) ) ;
#22112=LINE ( 'NONE', #1709, #19843 ) ;
#22163=DIRECTION ( 'NONE',  ( 0.000000000000000000, 0.000000000000000000, 1.000000000000000000 ) ) ;
#22171=VERTEX_POINT ( 'NONE', #58287 ) ;
#22177=ORIENTED_EDGE ( 'NONE', *, *, #29514, .F. ) ;
#22274=FACE_OUTER_BOUND ( 'NONE', #62000, .T. ) ;
#22300=AXIS2_PLACEMENT_3D ( 'NONE', #67300, #40204, #50411 ) ;
#22333=CARTESIAN_POINT ( 'NONE',  ( 123.4242852856285566, 10.00000000000000000, -30.00000000000000000 ) ) ;
#22427=ORIENTED_EDGE ( 'NONE', *, *, #59840, .T. ) ;
#22434=VERTEX_POINT ( 'NONE', #52588 ) ;
#22460=DIRECTION ( 'NONE',  ( -0.000000000000000000, -1.000000000000000000, -0.000000000000000000 ) ) ;
#22507=DIRECTION ( 'NONE',  ( 0.000000000000000000, 0.000000000000000000, -1.000000000000000000 ) ) ;
#22515=VECTOR ( 'NONE', #21948, 1000.000000000000000 ) ;
#22623=DIRECTION ( 'NONE',  ( 0.000000000000000000, 1.000000000000000000, 0.000000000000000000 ) ) ;
#22686=ORIENTED_EDGE ( 'NONE', *, *, #34348, .F. ) ;
#22758=ORIENTED_EDGE ( 'NONE', *, *, #30250, .T. ) ;
#22862=DIRECTION ( 'NONE',  ( -0.7071067811865474617, 0.000000000000000000, 0.7071067811865474617 ) ) ;
#22863=AXIS2_PLACEMENT_3D ( 'NONE', #60797, #7701, #55171 ) ;
#22936=FACE_OUTER_BOUND ( 'NONE', #60123, .T. ) ;
#22965=ORIENTED_EDGE ( 'NONE', *, *, #7165, .T. ) ;
#22979=DIRECTION ( 'NONE',  ( -1.000000000000000000, 0.000000000000000000, -0.000000000000000000 ) ) ;
#23024=LINE ( 'NONE', #23390, #45267 ) ;
#23037=DIRECTION ( 'NONE',  ( 0.000000000000000000, 0.000000000000000000, -1.000000000000000000 ) ) ;
#23191=VERTEX_POINT ( 'NONE', #59073 ) ;
#23234=ORIENTED_EDGE ( 'NONE', *, *, #48567, .F. ) ;
#23319=FACE_OUTER_BOUND ( 'NONE', #68966, .T. ) ;
#23390=CARTESIAN_POINT ( 'NONE',  ( 196.9999999999999716, 6.000000000000000000, 0.000000000000000000 ) ) ;
#23391=DIRECTION ( 'NONE',  ( 0.000000000000000000, 0.000000000000000000, -1.000000000000000000 ) ) ;
#23399=DIRECTION ( 'NONE',  ( -0.000000000000000000, -1.000000000000000000, -0.000000000000000000 ) ) ;
#23409=CARTESIAN_POINT ( 'NONE',  ( 196.9999999999999716, 6.000000000000000000, 0.000000000000000000 ) ) ;
#23477=CARTESIAN_POINT ( 'NONE',  ( 50.97490815085634352, 6.000000000000000000, -9.435653166495500344 ) ) ;
#23505=ORIENTED_EDGE ( 'NONE', *, *, #4432, .T. ) ;
#23519=DIRECTION ( 'NONE',  ( 1.000000000000000000, 0.000000000000000000, 0.000000000000000000 ) ) ;
#23531=EDGE_CURVE ( 'NONE', #32688, #41760, #52189, .T. ) ;
#23537=EDGE_CURVE ( 'NONE', #21697, #34571, #7553, .T. ) ;
#23638=CARTESIAN_POINT ( 'NONE',  ( 123.4242852856285566, 0.000000000000000000, -30.00000000000000000 ) ) ;
#23719=FILL_AREA_STYLE ('',( #66996 ) ) ;
#23754=DIRECTION ( 'NONE',  ( -0.000000000000000000, 0.7071067811865474617, 0.7071067811865474617 ) ) ;
#24181=AXIS2_PLACEMENT_3D ( 'NONE', #30663, #24704, #31020 ) ;
#24201=DIRECTION ( 'NONE',  ( 0.000000000000000000, 0.000000000000000000, 1.000000000000000000 ) ) ;
#24215=DIRECTION ( 'NONE',  ( 0.000000000000000000, 0.000000000000000000, -1.000000000000000000 ) ) ;
#24285=PRODUCT_DEFINITION_FORMATION_WITH_SPECIFIED_SOURCE ( 'ANY', '', #67620, .NOT_KNOWN. ) ;
#24292=DIRECTION ( 'NONE',  ( 0.000000000000000000, -0.7071067811865474617, 0.7071067811865474617 ) ) ;
#24383=AXIS2_PLACEMENT_3D ( 'NONE', #16842, #11216, #32683 ) ;
#24430=CIRCLE ( 'NONE', #1982, 5.000000000000018652 ) ;
#24467=VECTOR ( 'NONE', #1239, 1000.000000000000114 ) ;
#24486=EDGE_CURVE ( 'NONE', #17220, #10774, #9513, .T. ) ;
#24532=CARTESIAN_POINT ( 'NONE',  ( 50.97490815085634352, 0.000000000000000000, -9.435653166495500344 ) ) ;
#24533=AXIS2_PLACEMENT_3D ( 'NONE', #48863, #11246, #22163 ) ;
#24683=FACE_OUTER_BOUND ( 'NONE', #10543, .T. ) ;
#24704=DIRECTION ( 'NONE',  ( 0.5773502691896258421, 0.5773502691896258421, -0.5773502691896258421 ) ) ;
#24839=ORIENTED_EDGE ( 'NONE', *, *, #67334, .T. ) ;
#24882=DIRECTION ( 'NONE',  ( -0.000000000000000000, -1.000000000000000000, -0.000000000000000000 ) ) ;
#24973=ADVANCED_FACE ( 'NONE', ( #28300 ), #38870, .F. ) ;
#25019=EDGE_CURVE ( 'NONE', #66403, #30796, #66316, .T. ) ;
#25026=DIRECTION ( 'NONE',  ( 1.000000000000000000, 0.000000000000000000, 0.000000000000000000 ) ) ;
#25059=ORIENTED_EDGE ( 'NONE', *, *, #7324, .F. ) ;
#25131=ORIENTED_EDGE ( 'NONE', *, *, #7779, .T. ) ;
#25136=DIRECTION ( 'NONE',  ( -1.000000000000000000, 0.000000000000000000, 0.000000000000000000 ) ) ;
#25149=AXIS2_PLACEMENT_3D ( 'NONE', #21215, #58830, #14889 ) ;
#25175=CARTESIAN_POINT ( 'NONE',  ( 76.57571471437145760, 0.000000000000000000, -20.00000000000000000 ) ) ;
#25183=CIRCLE ( 'NONE', #6015, 4.999999999999997335 ) ;
#25501=DIRECTION ( 'NONE',  ( 0.5773502691896258421, -0.5773502691896258421, 0.5773502691896258421 ) ) ;
#25510=FACE_BOUND ( 'NONE', #4101, .T. ) ;
#25548=CARTESIAN_POINT ( 'NONE',  ( 123.4242852856285566, 0.000000000000000000, -20.00000000000000000 ) ) ;
#25561=CARTESIAN_POINT ( 'NONE',  ( 50.97490815085634352, 0.000000000000000000, -41.68900338898716740 ) ) ;
#25584=FACE_OUTER_BOUND ( 'NONE', #9045, .T. ) ;
#25659=EDGE_CURVE ( 'NONE', #9838, #7089, #30309, .T. ) ;
#25664=CARTESIAN_POINT ( 'NONE',  ( 183.2136430849848239, 0.000000000000000000, -9.435653166495541200 ) ) ;
#25673=CIRCLE ( 'NONE', #20040, 5.000000000000000888 ) ;
#25704=ORIENTED_EDGE ( 'NONE', *, *, #62580, .T. ) ;
#25707=ORIENTED_EDGE ( 'NONE', *, *, #31739, .F. ) ;
#25736=EDGE_CURVE ( 'NONE', #56977, #1254, #16191, .T. ) ;
#25742=PLANE ( 'NONE',  #24181 ) ;
#25842=PLANE ( 'NONE',  #8518 ) ;
#25957=EDGE_CURVE ( 'NONE', #30445, #50693, #63586, .T. ) ;
#26010=CARTESIAN_POINT ( 'NONE',  ( 0.000000000000000000, 3.000000000000030198, 0.000000000000000000 ) ) ;
#26095=CARTESIAN_POINT ( 'NONE',  ( 149.0250918491436778, 6.000000000000000000, -14.43565316649551811 ) ) ;
#26380=PLANE ( 'NONE',  #24383 ) ;
#26395=VECTOR ( 'NONE', #69234, 1000.000000000000000 ) ;
#26403=DIRECTION ( 'NONE',  ( -1.000000000000000000, 0.000000000000000000, -1.734723475976805517E-15 ) ) ;
#26434=DIRECTION ( 'NONE',  ( -0.000000000000000000, -1.000000000000000000, -0.000000000000000000 ) ) ;
#26457=DIRECTION ( 'NONE',  ( -0.000000000000000000, -1.000000000000000000, -0.000000000000000000 ) ) ;
#26545=ADVANCED_FACE ( 'NONE', ( #67960 ), #25742, .T. ) ;
#26573=FACE_OUTER_BOUND ( 'NONE', #36664, .T. ) ;
#26582=AXIS2_PLACEMENT_3D ( 'NONE', #36904, #68231, #42176 ) ;
#26686=ADVANCED_FACE ( 'NONE', ( #57760 ), #15193, .F. ) ;
#26726=LINE ( 'NONE', #65050, #37570 ) ;
#26734=AXIS2_PLACEMENT_3D ( 'NONE', #12098, #11042, #33211 ) ;
#26767=ORIENTED_EDGE ( 'NONE', *, *, #50744, .F. ) ;
#26790=EDGE_CURVE ( 'NONE', #34571, #45847, #7064, .T. ) ;
#26842=ORIENTED_EDGE ( 'NONE', *, *, #25736, .T. ) ;
#26866=ORIENTED_EDGE ( 'NONE', *, *, #51543, .F. ) ;
#26884=DIRECTION ( 'NONE',  ( 0.000000000000000000, -1.000000000000000000, 0.000000000000000000 ) ) ;
#26914=AXIS2_PLACEMENT_3D ( 'NONE', #25561, #14305, #40337 ) ;
#26933=EDGE_LOOP ( 'NONE', ( #3694, #23505, #37821, #60412 ) ) ;
#26952=ORIENTED_EDGE ( 'NONE', *, *, #31156, .F. ) ;
#26989=ORIENTED_EDGE ( 'NONE', *, *, #6166, .F. ) ;
#27062=EDGE_CURVE ( 'NONE', #10488, #18148, #1008, .T. ) ;
#27074=CARTESIAN_POINT ( 'NONE',  ( 149.0250918491436778, 6.000000000000000000, -4.435653166495538535 ) ) ;
#27114=VECTOR ( 'NONE', #2616, 1000.000000000000114 ) ;
#27184=CLOSED_SHELL ( 'NONE', ( #24973, #17151, #68702, #54270, #30981, #9457, #11328, #37451, #19224, #44858, #13301, #69305, #28429, #1207, #35836, #35349, #26686, #57261, #12223, #67538, #9380, #69481, #31758, #36687, #43403, #10542, #66011, #36763, #44521, #42877, #26545, #57743, #17375, #36957, #32405, #39442, #11987, #43506, #50980, #19545, #63721, #4601, #55821, #61105, #51052 ) ) ;
#27196=CARTESIAN_POINT ( 'NONE',  ( 200.0000000000000000, 3.000000000000030198, -46.99999999999997158 ) ) ;
#27209=FACE_OUTER_BOUND ( 'NONE', #47502, .T. ) ;
#27212=CARTESIAN_POINT ( 'NONE',  ( 196.9999999999999716, 6.000000000000000000, -46.99999999999997158 ) ) ;
#27230=EDGE_CURVE ( 'NONE', #56047, #22100, #50075, .T. ) ;
#27259=DIRECTION ( 'NONE',  ( 0.000000000000000000, 0.000000000000000000, -1.000000000000000000 ) ) ;
#27291=FACE_OUTER_BOUND ( 'NONE', #9591, .T. ) ;
#27356=CARTESIAN_POINT ( 'NONE',  ( 50.97490815085634352, 0.000000000000000000, -46.68900338898716029 ) ) ;
#27365=CIRCLE ( 'NONE', #66730, 5.000000000000000888 ) ;
#27398=DIRECTION ( 'NONE',  ( -0.000000000000000000, -1.000000000000000000, -0.000000000000000000 ) ) ;
#27414=VERTEX_POINT ( 'NONE', #44442 ) ;
#27419=AXIS2_PLACEMENT_3D ( 'NONE', #55017, #18098, #23391 ) ;
#27488=DIRECTION ( 'NONE',  ( -0.000000000000000000, -1.000000000000000000, -0.000000000000000000 ) ) ;
#27560=FACE_OUTER_BOUND ( 'NONE', #53483, .T. ) ;
#27577=CARTESIAN_POINT ( 'NONE',  ( 3.000000000000028866, 0.000000000000000000, -3.000000000000030198 ) ) ;
#27593=DIRECTION ( 'NONE',  ( 0.000000000000000000, 0.000000000000000000, 1.000000000000000000 ) ) ;
#27658=ORIENTED_EDGE ( 'NONE', *, *, #35893, .F. ) ;
#27682=DIRECTION ( 'NONE',  ( 0.000000000000000000, 0.000000000000000000, -1.000000000000000000 ) ) ;
#27701=CARTESIAN_POINT ( 'NONE',  ( 3.000000000000004441, 3.000000000000030198, -50.00000000000000000 ) ) ;
#27723=LINE ( 'NONE', #6972, #11157 ) ;
#27792=ORIENTED_EDGE ( 'NONE', *, *, #32326, .F. ) ;
#27816=VECTOR ( 'NONE', #59261, 1000.000000000000000 ) ;
#27947=EDGE_CURVE ( 'NONE', #11659, #5640, #38656, .T. ) ;
#27963=CARTESIAN_POINT ( 'NONE',  ( 0.000000000000000000, 2.999999999999969358, 0.000000000000000000 ) ) ;
#28180=VECTOR ( 'NONE', #50707, 1000.000000000000000 ) ;
#28240=DIRECTION ( 'NONE',  ( 0.000000000000000000, 0.000000000000000000, -1.000000000000000000 ) ) ;
#28243=VERTEX_POINT ( 'NONE', #56220 ) ;
#28245=ORIENTED_EDGE ( 'NONE', *, *, #60338, .F. ) ;
#28256=ORIENTED_EDGE ( 'NONE', *, *, #28514, .F. ) ;
#28257=FACE_BOUND ( 'NONE', #45978, .T. ) ;
#28290=DIRECTION ( 'NONE',  ( 0.000000000000000000, 0.000000000000000000, 1.000000000000000000 ) ) ;
#28300=FACE_OUTER_BOUND ( 'NONE', #29854, .T. ) ;
#28311=DIRECTION ( 'NONE',  ( -5.551115123125781716E-16, 0.000000000000000000, -1.000000000000000000 ) ) ;
#28429=ADVANCED_FACE ( 'NONE', ( #21693 ), #32945, .F. ) ;
#28453=DIRECTION ( 'NONE',  ( 0.000000000000000000, 0.000000000000000000, 1.000000000000000000 ) ) ;
#28514=EDGE_CURVE ( 'NONE', #10774, #12136, #39622, .T. ) ;
#28582=PLANE ( 'NONE',  #4941 ) ;
#28620=ORIENTED_EDGE ( 'NONE', *, *, #37114, .T. ) ;
#28621=LINE ( 'NONE', #44798, #66632 ) ;
#28648=SURFACE_SIDE_STYLE ('',( #45162 ) ) ;
#28673=CARTESIAN_POINT ( 'NONE',  ( 50.97490815085634352, 6.000000000000000000, -46.68900338898716029 ) ) ;
#28716=LINE ( 'NONE', #1626, #3410 ) ;
#28736=DIRECTION ( 'NONE',  ( 0.000000000000000000, 0.000000000000000000, -1.000000000000000000 ) ) ;
#28804=ORIENTED_EDGE ( 'NONE', *, *, #31739, .T. ) ;
#28848=CARTESIAN_POINT ( 'NONE',  ( 196.9999999999999716, 2.999999999999969802, 0.000000000000000000 ) ) ;
#28902=LINE ( 'NONE', #40143, #63392 ) ;
#28931=LINE ( 'NONE', #6420, #69245 ) ;
#28951=DIRECTION ( 'NONE',  ( -0.000000000000000000, -1.000000000000000000, -0.000000000000000000 ) ) ;
#29009=CARTESIAN_POINT ( 'NONE',  ( 196.9999999999999716, 0.000000000000000000, -3.000000000000030198 ) ) ;
#29025=CARTESIAN_POINT ( 'NONE',  ( 50.97490815085634352, 6.000000000000000000, -14.43565316649549679 ) ) ;
#29028=EDGE_LOOP ( 'NONE', ( #36390, #56034 ) ) ;
#29098=DIRECTION ( 'NONE',  ( -0.000000000000000000, -1.000000000000000000, -0.000000000000000000 ) ) ;
#29170=ORIENTED_EDGE ( 'NONE', *, *, #44240, .F. ) ;
#29178=FACE_OUTER_BOUND ( 'NONE', #19176, .T. ) ;
#29212=LINE ( 'NONE', #39413, #30056 ) ;
#29244=EDGE_LOOP ( 'NONE', ( #61381, #40740, #50249, #29170 ) ) ;
#29251=AXIS2_PLACEMENT_3D ( 'NONE', #14946, #26884, #31476 ) ;
#29348=CARTESIAN_POINT ( 'NONE',  ( 99.99999999999997158, 6.000000000000000000, -46.99999999999998579 ) ) ;
#29363=LINE ( 'NONE', #19150, #49510 ) ;
#29368=PLANE ( 'NONE',  #64063 ) ;
#29487=ORIENTED_EDGE ( 'NONE', *, *, #7324, .T. ) ;
#29490=CARTESIAN_POINT ( 'NONE',  ( 121.4242852856285140, 0.000000000000000000, -20.00000000000000000 ) ) ;
#29514=EDGE_CURVE ( 'NONE', #22434, #40256, #45601, .T. ) ;
#29515=CARTESIAN_POINT ( 'NONE',  ( 50.97490815085634352, 6.000000000000000000, -36.68900338898716740 ) ) ;
#29532=AXIS2_PLACEMENT_3D ( 'NONE', #31726, #10607, #4646 ) ;
#29540=ORIENTED_EDGE ( 'NONE', *, *, #68607, .T. ) ;
#29567=ORIENTED_EDGE ( 'NONE', *, *, #34348, .T. ) ;
#29588=CARTESIAN_POINT ( 'NONE',  ( 123.4242852856285566, 6.000000000000000000, -30.00000000000000000 ) ) ;
#29595=CIRCLE ( 'NONE', #64383, 21.99999999999998579 ) ;
#29611=ORIENTED_EDGE ( 'NONE', *, *, #32716, .F. ) ;
#29627=DIRECTION ( 'NONE',  ( 0.000000000000000000, 1.000000000000000000, 0.000000000000000000 ) ) ;
#29854=EDGE_LOOP ( 'NONE', ( #22758, #32519, #20518, #57717 ) ) ;
#29878=ORIENTED_EDGE ( 'NONE', *, *, #39464, .F. ) ;
#29908=ORIENTED_EDGE ( 'NONE', *, *, #25019, .T. ) ;
#29936=CARTESIAN_POINT ( 'NONE',  ( 123.4242852856285566, 0.000000000000000000, -30.00000000000000000 ) ) ;
#30022=ORIENTED_EDGE ( 'NONE', *, *, #62986, .T. ) ;
#30037=PRESENTATION_STYLE_ASSIGNMENT (( #18785 ) ) ;
#30056=VECTOR ( 'NONE', #51016, 1000.000000000000000 ) ;
#30102=VECTOR ( 'NONE', #23754, 1000.000000000000114 ) ;
#30123=SHAPE_REPRESENTATION_RELATIONSHIP ( 'NONE' , 'NONE' ,  #34334, #41606 ) ;
#30164=CARTESIAN_POINT ( 'NONE',  ( 16.78635691501517613, 6.000000000000000000, -9.435653166495500344 ) ) ;
#30206=VERTEX_POINT ( 'NONE', #16256 ) ;
#30250=EDGE_CURVE ( 'NONE', #63181, #40287, #24430, .T. ) ;
#30309=LINE ( 'NONE', #40858, #11862 ) ;
#30336=VERTEX_POINT ( 'NONE', #29588 ) ;
#30342=DIRECTION ( 'NONE',  ( 0.7071067811865475727, -0.7071067811865475727, -3.925231146709437301E-16 ) ) ;
#30395=EDGE_LOOP ( 'NONE', ( #29540, #42443, #39081 ) ) ;
#30414=FACE_OUTER_BOUND ( 'NONE', #20517, .T. ) ;
#30445=VERTEX_POINT ( 'NONE', #62654 ) ;
#30467=ORIENTED_EDGE ( 'NONE', *, *, #37316, .T. ) ;
#30496=CARTESIAN_POINT ( 'NONE',  ( 16.78635691501517613, 6.000000000000000000, -36.68900338898716740 ) ) ;
#30530=CARTESIAN_POINT ( 'NONE',  ( 16.78635691501517613, 6.000000000000000000, -4.435653166495499455 ) ) ;
#30561=AXIS2_PLACEMENT_3D ( 'NONE', #6617, #48805, #49504 ) ;
#30663=CARTESIAN_POINT ( 'NONE',  ( 200.0000000000000000, 2.999999999999969802, -46.99999999999997158 ) ) ;
#30796=VERTEX_POINT ( 'NONE', #62212 ) ;
#30937=ORIENTED_EDGE ( 'NONE', *, *, #14756, .F. ) ;
#30981=ADVANCED_FACE ( 'NONE', ( #2707 ), #13601, .F. ) ;
#30996=AXIS2_PLACEMENT_3D ( 'NONE', #31462, #8637, #3686 ) ;
#31011=EDGE_CURVE ( 'NONE', #41654, #30206, #39987, .T. ) ;
#31020=DIRECTION ( 'NONE',  ( -0.7071067811865475727, 0.000000000000000000, -0.7071067811865475727 ) ) ;
#31037=LINE ( 'NONE', #36309, #31173 ) ;
#31065=ORIENTED_EDGE ( 'NONE', *, *, #50300, .T. ) ;
#31129=FACE_OUTER_BOUND ( 'NONE', #39169, .T. ) ;
#31156=EDGE_CURVE ( 'NONE', #63882, #42425, #37815, .T. ) ;
#31173=VECTOR ( 'NONE', #40540, 1000.000000000000000 ) ;
#31275=EDGE_CURVE ( 'NONE', #50282, #50676, #45177, .T. ) ;
#31375=DIRECTION ( 'NONE',  ( -0.000000000000000000, -1.000000000000000000, -0.000000000000000000 ) ) ;
#31431=ORIENTED_EDGE ( 'NONE', *, *, #56947, .T. ) ;
#31462=CARTESIAN_POINT ( 'NONE',  ( 0.000000000000000000, 0.000000000000000000, 0.000000000000000000 ) ) ;
#31476=DIRECTION ( 'NONE',  ( 0.000000000000000000, 0.000000000000000000, -1.000000000000000000 ) ) ;
#31573=ORIENTED_EDGE ( 'NONE', *, *, #59840, .F. ) ;
#31594=EDGE_CURVE ( 'NONE', #28243, #43052, #57107, .T. ) ;
#31622=CYLINDRICAL_SURFACE ( 'NONE', #26582, 4.999999999999990230 ) ;
#31651=AXIS2_PLACEMENT_3D ( 'NONE', #10224, #47501, #68961 ) ;
#31726=CARTESIAN_POINT ( 'NONE',  ( 200.0000000000000000, 3.000000000000030198, 0.000000000000000000 ) ) ;
#31734=EDGE_CURVE ( 'NONE', #22434, #21697, #66145, .T. ) ;
#31739=EDGE_CURVE ( 'NONE', #66403, #62711, #33512, .T. ) ;
#31758=ADVANCED_FACE ( 'NONE', ( #39048 ), #1056, .F. ) ;
#31811=VERTEX_POINT ( 'NONE', #35848 ) ;
#31856=CIRCLE ( 'NONE', #19455, 4.999999999999996447 ) ;
#31872=ORIENTED_EDGE ( 'NONE', *, *, #31594, .F. ) ;
#31891=CARTESIAN_POINT ( 'NONE',  ( 0.000000000000000000, 6.000000000000000000, 0.000000000000000000 ) ) ;
#32000=EDGE_CURVE ( 'NONE', #22100, #35032, #64998, .T. ) ;
#32011=AXIS2_PLACEMENT_3D ( 'NONE', #25664, #4537, #46060 ) ;
#32140=CARTESIAN_POINT ( 'NONE',  ( 123.4242852856285566, 0.000000000000000000, -20.00000000000000000 ) ) ;
#32189=CARTESIAN_POINT ( 'NONE',  ( 200.0000000000000000, 2.999999999999969802, 0.000000000000000000 ) ) ;
#32199=SHAPE_DEFINITION_REPRESENTATION ( #17578, #34334 ) ;
#32231=ORIENTED_EDGE ( 'NONE', *, *, #50505, .T. ) ;
#32326=EDGE_CURVE ( 'NONE', #3913, #5640, #50124, .T. ) ;
#32405=ADVANCED_FACE ( 'NONE', ( #17772 ), #11085, .F. ) ;
#32425=VERTEX_POINT ( 'NONE', #53978 ) ;
#32519=ORIENTED_EDGE ( 'NONE', *, *, #34342, .T. ) ;
#32563=CARTESIAN_POINT ( 'NONE',  ( 149.0250918491436494, 6.000000000000000000, -46.68900338898718161 ) ) ;
#32576=CARTESIAN_POINT ( 'NONE',  ( 123.4242852856285566, 6.000000000000000000, -20.00000000000000000 ) ) ;
#32683=DIRECTION ( 'NONE',  ( -1.000000000000000000, 0.000000000000000000, 0.000000000000000000 ) ) ;
#32688=VERTEX_POINT ( 'NONE', #58492 ) ;
#32716=EDGE_CURVE ( 'NONE', #51453, #22434, #36368, .T. ) ;
#32776=FACE_OUTER_BOUND ( 'NONE', #34262, .T. ) ;
#32877=DIRECTION ( 'NONE',  ( 0.000000000000000000, 1.000000000000000000, 0.000000000000000000 ) ) ;
#32945=CYLINDRICAL_SURFACE ( 'NONE', #34377, 21.99999999999998579 ) ;
#33036=LINE ( 'NONE', #16845, #64100 ) ;
#33066=CARTESIAN_POINT ( 'NONE',  ( 196.9999999999999716, 6.000000000000000000, -3.000000000000030198 ) ) ;
#33093=PLANE ( 'NONE',  #64574 ) ;
#33103=CARTESIAN_POINT ( 'NONE',  ( 76.57571471437145760, 0.000000000000000000, -30.00000000000000000 ) ) ;
#33211=DIRECTION ( 'NONE',  ( 0.000000000000000000, 0.000000000000000000, -1.000000000000000000 ) ) ;
#33248=DIRECTION ( 'NONE',  ( -1.734723475976805517E-15, 0.000000000000000000, 1.000000000000000000 ) ) ;
#33333=CYLINDRICAL_SURFACE ( 'NONE', #43032, 5.000000000000018652 ) ;
#33445=EDGE_CURVE ( 'NONE', #30796, #45847, #1109, .T. ) ;
#33456=CARTESIAN_POINT ( 'NONE',  ( 16.78635691501517613, 0.000000000000000000, -41.68900338898716740 ) ) ;
#33512=CIRCLE ( 'NONE', #58198, 21.99999999999998579 ) ;
#33519=AXIS2_PLACEMENT_3D ( 'NONE', #43718, #38818, #54978 ) ;
#33632=DIRECTION ( 'NONE',  ( -5.551115123125781716E-16, 0.000000000000000000, -1.000000000000000000 ) ) ;
#33747=ORIENTED_EDGE ( 'NONE', *, *, #34300, .T. ) ;
#33771=ORIENTED_EDGE ( 'NONE', *, *, #41333, .F. ) ;
#33784=CIRCLE ( 'NONE', #58467, 21.99999999999998579 ) ;
#33814=ORIENTED_EDGE ( 'NONE', *, *, #60180, .T. ) ;
#34045=ORIENTED_EDGE ( 'NONE', *, *, #36081, .T. ) ;
#34051=DIRECTION ( 'NONE',  ( 0.000000000000000000, 1.000000000000000000, 0.000000000000000000 ) ) ;
#34118=STYLED_ITEM ( 'NONE', ( #30037 ), #41410 ) ;
#34127=CIRCLE ( 'NONE', #22863, 4.999999999999997335 ) ;
#34153=DIRECTION ( 'NONE',  ( 0.000000000000000000, 0.000000000000000000, -1.000000000000000000 ) ) ;
#34262=EDGE_LOOP ( 'NONE', ( #22427, #31431, #17283, #59089 ) ) ;
#34264=EDGE_LOOP ( 'NONE', ( #17482, #61432 ) ) ;
#34300=EDGE_CURVE ( 'NONE', #66403, #11659, #27723, .T. ) ;
#34334=SHAPE_REPRESENTATION ( 'cutting blade', ( #66832 ), #6181 ) ;
#34342=EDGE_CURVE ( 'NONE', #40287, #32688, #38632, .T. ) ;
#34348=EDGE_CURVE ( 'NONE', #7089, #59608, #13985, .T. ) ;
#34377=AXIS2_PLACEMENT_3D ( 'NONE', #37527, #16424, #54388 ) ;
#34571=VERTEX_POINT ( 'NONE', #5496 ) ;
#34574=ORIENTED_EDGE ( 'NONE', *, *, #25659, .T. ) ;
#34596=EDGE_LOOP ( 'NONE', ( #46212, #40074 ) ) ;
#34665=DIRECTION ( 'NONE',  ( 0.000000000000000000, -0.7071067811865475727, 0.7071067811865475727 ) ) ;
#34762=ORIENTED_EDGE ( 'NONE', *, *, #7165, .F. ) ;
#35032=VERTEX_POINT ( 'NONE', #2839 ) ;
#35035=ORIENTED_EDGE ( 'NONE', *, *, #18126, .F. ) ;
#35116=DIRECTION ( 'NONE',  ( 0.000000000000000000, 1.000000000000000000, -0.000000000000000000 ) ) ;
#35144=DIRECTION ( 'NONE',  ( -0.000000000000000000, -1.000000000000000000, -0.000000000000000000 ) ) ;
#35167=ORIENTED_EDGE ( 'NONE', *, *, #64875, .T. ) ;
#35332=VECTOR ( 'NONE', #45370, 1000.000000000000000 ) ;
#35348=CARTESIAN_POINT ( 'NONE',  ( 99.99999999999997158, 0.000000000000000000, -25.00000000000000000 ) ) ;
#35349=ADVANCED_FACE ( 'NONE', ( #14350 ), #19617, .F. ) ;
#35432=VECTOR ( 'NONE', #10012, 1000.000000000000000 ) ;
#35443=CARTESIAN_POINT ( 'NONE',  ( 123.4242852856285566, 0.000000000000000000, -20.00000000000000000 ) ) ;
#35447=ORIENTED_EDGE ( 'NONE', *, *, #6166, .T. ) ;
#35571=EDGE_LOOP ( 'NONE', ( #36212, #11586, #14482, #47785 ) ) ;
#35786=DIRECTION ( 'NONE',  ( 0.000000000000000000, 0.000000000000000000, -1.000000000000000000 ) ) ;
#35805=DIRECTION ( 'NONE',  ( -0.000000000000000000, -1.000000000000000000, -0.000000000000000000 ) ) ;
#35836=ADVANCED_FACE ( 'NONE', ( #5431, #21601, #37094, #20564, #63488 ), #10024, .T. ) ;
#35848=CARTESIAN_POINT ( 'NONE',  ( 99.99999999999997158, 0.000000000000000000, -3.000000000000030198 ) ) ;
#35855=AXIS2_PLACEMENT_3D ( 'NONE', #31891, #13810, #60356 ) ;
#35893=EDGE_CURVE ( 'NONE', #1254, #66403, #59567, .T. ) ;
#35959=CARTESIAN_POINT ( 'NONE',  ( 50.97490815085634352, 6.000000000000000000, -41.68900338898716740 ) ) ;
#36019=ORIENTED_EDGE ( 'NONE', *, *, #57827, .F. ) ;
#36081=EDGE_CURVE ( 'NONE', #18148, #53590, #6843, .T. ) ;
#36212=ORIENTED_EDGE ( 'NONE', *, *, #48567, .T. ) ;
#36213=FACE_OUTER_BOUND ( 'NONE', #17584, .T. ) ;
#36246=EDGE_LOOP ( 'NONE', ( #41938, #45628, #62585, #22177 ) ) ;
#36269=AXIS2_PLACEMENT_3D ( 'NONE', #24532, #14313, #41393 ) ;
#36309=CARTESIAN_POINT ( 'NONE',  ( 0.000000000000000000, 0.000000000000000000, -3.000000000000030198 ) ) ;
#36353=DIRECTION ( 'NONE',  ( 0.000000000000000000, 0.000000000000000000, -1.000000000000000000 ) ) ;
#36368=LINE ( 'NONE', #62760, #44847 ) ;
#36390=ORIENTED_EDGE ( 'NONE', *, *, #68300, .T. ) ;
#36435=VECTOR ( 'NONE', #59017, 1000.000000000000000 ) ;
#36476=VERTEX_POINT ( 'NONE', #43757 ) ;
#36503=DIRECTION ( 'NONE',  ( -0.000000000000000000, -1.000000000000000000, -0.000000000000000000 ) ) ;
#36645=EDGE_CURVE ( 'NONE', #59608, #27414, #51060, .T. ) ;
#36664=EDGE_LOOP ( 'NONE', ( #55707, #49282, #44542, #65724 ) ) ;
#36687=ADVANCED_FACE ( 'NONE', ( #22936 ), #66560, .T. ) ;
#36707=FACE_OUTER_BOUND ( 'NONE', #52716, .T. ) ;
#36763=ADVANCED_FACE ( 'NONE', ( #24683 ), #68281, .T. ) ;
#36778=CIRCLE ( 'NONE', #50290, 5.000000000000000888 ) ;
#36904=CARTESIAN_POINT ( 'NONE',  ( 149.0250918491436778, 6.000000000000000000, -9.435653166495526989 ) ) ;
#36957=ADVANCED_FACE ( 'NONE', ( #29178 ), #2441, .F. ) ;
#36958=CARTESIAN_POINT ( 'NONE',  ( 76.57571471437145760, 10.00000000000000000, -30.00000000000000000 ) ) ;
#37079=EDGE_CURVE ( 'NONE', #9838, #30336, #44481, .T. ) ;
#37094=FACE_BOUND ( 'NONE', #42854, .T. ) ;
#37114=EDGE_CURVE ( 'NONE', #56047, #8968, #878, .T. ) ;
#37125=ORIENTED_EDGE ( 'NONE', *, *, #64901, .T. ) ;
#37220=AXIS2_PLACEMENT_3D ( 'NONE', #47054, #36503, #9085 ) ;
#37237=ORIENTED_EDGE ( 'NONE', *, *, #27230, .F. ) ;
#37316=EDGE_CURVE ( 'NONE', #50492, #64271, #55374, .T. ) ;
#37451=ADVANCED_FACE ( 'NONE', ( #36707 ), #14887, .F. ) ;
#37505=ORIENTED_EDGE ( 'NONE', *, *, #7716, .F. ) ;
#37527=CARTESIAN_POINT ( 'NONE',  ( 99.99999999999997158, 6.000000000000000000, -25.00000000000000000 ) ) ;
#37533=DIRECTION ( 'NONE',  ( -0.000000000000000000, -1.000000000000000000, -0.000000000000000000 ) ) ;
#37557=DIRECTION ( 'NONE',  ( -0.000000000000000000, -1.000000000000000000, -0.000000000000000000 ) ) ;
#37570=VECTOR ( 'NONE', #38307, 1000.000000000000114 ) ;
#37710=CARTESIAN_POINT ( 'NONE',  ( 183.2136430849847955, 6.000000000000000000, -41.68900338898720292 ) ) ;
#37815=LINE ( 'NONE', #60662, #27816 ) ;
#37821=ORIENTED_EDGE ( 'NONE', *, *, #21999, .F. ) ;
#37835=CARTESIAN_POINT ( 'NONE',  ( 76.57571471437145760, 10.00000000000000000, -20.00000000000000000 ) ) ;
#38130=EDGE_LOOP ( 'NONE', ( #8143, #18506, #7685, #53121 ) ) ;
#38251=ORIENTED_EDGE ( 'NONE', *, *, #25659, .F. ) ;
#38300=CARTESIAN_POINT ( 'NONE',  ( 1.499999999999989564, 4.499999999999984901, -46.99999999999997158 ) ) ;
#38307=DIRECTION ( 'NONE',  ( 0.7071067811865474617, 0.7071067811865474617, -0.000000000000000000 ) ) ;
#38320=PRODUCT_DEFINITION ( 'UNKNOWN', '', #24285, #64797 ) ;
#38456=CARTESIAN_POINT ( 'NONE',  ( -5.204170427930393515E-14, 6.000000000000000000, -29.99999999999986855 ) ) ;
#38478=DIRECTION ( 'NONE',  ( 0.000000000000000000, 0.000000000000000000, -1.000000000000000000 ) ) ;
#38511=DIRECTION ( 'NONE',  ( -0.000000000000000000, -1.000000000000000000, -0.000000000000000000 ) ) ;
#38578=CYLINDRICAL_SURFACE ( 'NONE', #57817, 4.999999999999990230 ) ;
#38583=AXIS2_PLACEMENT_3D ( 'NONE', #52067, #8824, #46434 ) ;
#38611=EDGE_CURVE ( 'NONE', #43052, #28243, #10396, .T. ) ;
#38632=LINE ( 'NONE', #11893, #52727 ) ;
#38656=LINE ( 'NONE', #38300, #21996 ) ;
#38680=ORIENTED_EDGE ( 'NONE', *, *, #54016, .T. ) ;
#38775=DIRECTION ( 'NONE',  ( 0.000000000000000000, 1.000000000000000000, 0.000000000000000000 ) ) ;
#38813=LINE ( 'NONE', #38456, #1740 ) ;
#38818=DIRECTION ( 'NONE',  ( 0.000000000000000000, 1.000000000000000000, -0.000000000000000000 ) ) ;
#38868=DIRECTION ( 'NONE',  ( -0.000000000000000000, -1.000000000000000000, -0.000000000000000000 ) ) ;
#38870=CYLINDRICAL_SURFACE ( 'NONE', #41044, 5.000000000000018652 ) ;
#38932=CARTESIAN_POINT ( 'NONE',  ( 16.78635691501517613, 0.000000000000000000, -9.435653166495500344 ) ) ;
#39048=FACE_OUTER_BOUND ( 'NONE', #41047, .T. ) ;
#39081=ORIENTED_EDGE ( 'NONE', *, *, #69057, .F. ) ;
#39102=CYLINDRICAL_SURFACE ( 'NONE', #357, 5.000000000000018652 ) ;
#39123=LINE ( 'NONE', #779, #7220 ) ;
#39149=DIRECTION ( 'NONE',  ( 0.000000000000000000, 0.000000000000000000, 1.000000000000000000 ) ) ;
#39167=LINE ( 'NONE', #66599, #21956 ) ;
#39169=EDGE_LOOP ( 'NONE', ( #29567, #396, #30022, #17406, #55695, #50027, #11741, #33814 ) ) ;
#39207=( NAMED_UNIT ( * ) SI_UNIT ( $, .STERADIAN. ) SOLID_ANGLE_UNIT ( ) );
#39278=CARTESIAN_POINT ( 'NONE',  ( 183.2136430849847955, 6.000000000000000000, -36.68900338898718871 ) ) ;
#39297=DIRECTION ( 'NONE',  ( -0.000000000000000000, -1.000000000000000000, -0.000000000000000000 ) ) ;
#39366=CARTESIAN_POINT ( 'NONE',  ( 183.2136430849848239, 6.000000000000000000, -4.435653166495524324 ) ) ;
#39369=VERTEX_POINT ( 'NONE', #4315 ) ;
#39413=CARTESIAN_POINT ( 'NONE',  ( -2.775557561562891351E-14, 2.999999999999969802, -50.00000000000000000 ) ) ;
#39437=CARTESIAN_POINT ( 'NONE',  ( 3.000000000000004441, 6.000000000000000000, -46.99999999999997158 ) ) ;
#39438=LINE ( 'NONE', #17642, #49081 ) ;
#39442=ADVANCED_FACE ( 'NONE', ( #52495 ), #14855, .T. ) ;
#39449=CIRCLE ( 'NONE', #9124, 4.999999999999990230 ) ;
#39464=EDGE_CURVE ( 'NONE', #62549, #69370, #69002, .T. ) ;
#39507=ORIENTED_EDGE ( 'NONE', *, *, #6461, .T. ) ;
#39622=LINE ( 'NONE', #61424, #15326 ) ;
#39708=CARTESIAN_POINT ( 'NONE',  ( 99.99999999999997158, 0.000000000000000000, -25.00000000000000000 ) ) ;
#39865=EDGE_LOOP ( 'NONE', ( #48452, #64125, #12280 ) ) ;
#39871=DIRECTION ( 'NONE',  ( 0.000000000000000000, 1.000000000000000000, -0.000000000000000000 ) ) ;
#39940=AXIS2_PLACEMENT_3D ( 'NONE', #30164, #24882, #35786 ) ;
#39987=LINE ( 'NONE', #56504, #57059 ) ;
#40074=ORIENTED_EDGE ( 'NONE', *, *, #23531, .T. ) ;
#40143=CARTESIAN_POINT ( 'NONE',  ( 200.0000000000000000, 2.999999999999969802, -46.99999999999997158 ) ) ;
#40188=DIRECTION ( 'NONE',  ( 0.000000000000000000, 0.000000000000000000, 1.000000000000000000 ) ) ;
#40204=DIRECTION ( 'NONE',  ( 0.000000000000000000, 0.000000000000000000, 1.000000000000000000 ) ) ;
#40234=VECTOR ( 'NONE', #2451, 1000.000000000000000 ) ;
#40256=VERTEX_POINT ( 'NONE', #11474 ) ;
#40287=VERTEX_POINT ( 'NONE', #39278 ) ;
#40337=DIRECTION ( 'NONE',  ( 0.000000000000000000, 0.000000000000000000, 1.000000000000000000 ) ) ;
#40458=ORIENTED_EDGE ( 'NONE', *, *, #34342, .F. ) ;
#40459=AXIS2_PLACEMENT_3D ( 'NONE', #55347, #17008, #38478 ) ;
#40528=CARTESIAN_POINT ( 'NONE',  ( 99.99999999999997158, 0.000000000000000000, -25.00000000000000000 ) ) ;
#40540=DIRECTION ( 'NONE',  ( -1.000000000000000000, 0.000000000000000000, 0.000000000000000000 ) ) ;
#40587=AXIS2_PLACEMENT_3D ( 'NONE', #44663, #45347, #13011 ) ;
#40604=DIRECTION ( 'NONE',  ( 5.551115123125781716E-16, 0.000000000000000000, 1.000000000000000000 ) ) ;
#40697=ORIENTED_EDGE ( 'NONE', *, *, #25019, .F. ) ;
#40702=ORIENTED_EDGE ( 'NONE', *, *, #7779, .F. ) ;
#40740=ORIENTED_EDGE ( 'NONE', *, *, #41333, .T. ) ;
#40743=ORIENTED_EDGE ( 'NONE', *, *, #8530, .T. ) ;
#40756=AXIS2_PLACEMENT_3D ( 'NONE', #16662, #43390, #1902 ) ;
#40849=CIRCLE ( 'NONE', #57674, 5.000000000000018652 ) ;
#40851=VECTOR ( 'NONE', #22862, 1000.000000000000114 ) ;
#40858=CARTESIAN_POINT ( 'NONE',  ( 123.4242852856285566, 10.00000000000000000, -20.00000000000000000 ) ) ;
#40889=PLANE ( 'NONE',  #60424 ) ;
#40966=LINE ( 'NONE', #7587, #30102 ) ;
#41005=CIRCLE ( 'NONE', #53323, 4.999999999999997335 ) ;
#41044=AXIS2_PLACEMENT_3D ( 'NONE', #2282, #55026, #23037 ) ;
#41047=EDGE_LOOP ( 'NONE', ( #40458, #24839, #66252, #48348 ) ) ;
#41184=ORIENTED_EDGE ( 'NONE', *, *, #45812, .F. ) ;
#41289=DIRECTION ( 'NONE',  ( -0.000000000000000000, -1.000000000000000000, -0.000000000000000000 ) ) ;
#41333=EDGE_CURVE ( 'NONE', #56977, #50492, #6835, .T. ) ;
#41337=DIRECTION ( 'NONE',  ( -0.7071067811865475727, 0.000000000000000000, 0.7071067811865475727 ) ) ;
#41391=EDGE_LOOP ( 'NONE', ( #50909, #16874, #59195, #13882, #25131 ) ) ;
#41393=DIRECTION ( 'NONE',  ( 0.000000000000000000, 0.000000000000000000, 1.000000000000000000 ) ) ;
#41408=VERTEX_POINT ( 'NONE', #29009 ) ;
#41410=MANIFOLD_SOLID_BREP ( 'Mirror1', #27184 ) ;
#41447=DIRECTION ( 'NONE',  ( 0.000000000000000000, 0.000000000000000000, -1.000000000000000000 ) ) ;
#41574=ORIENTED_EDGE ( 'NONE', *, *, #50505, .F. ) ;
#41606=ADVANCED_BREP_SHAPE_REPRESENTATION ( '', ( #41410, #66832 ), #6181 ) ;
#41654=VERTEX_POINT ( 'NONE', #7466 ) ;
#41686=ORIENTED_EDGE ( 'NONE', *, *, #1260, .T. ) ;
#41742=APPLICATION_CONTEXT ( 'automotive_design' ) ;
#41760=VERTEX_POINT ( 'NONE', #56680 ) ;
#41782=EDGE_CURVE ( 'NONE', #30336, #22171, #21456, .T. ) ;
#41805=VERTEX_POINT ( 'NONE', #27074 ) ;
#41938=ORIENTED_EDGE ( 'NONE', *, *, #31734, .T. ) ;
#42015=LINE ( 'NONE', #15289, #35432 ) ;
#42088=EDGE_CURVE ( 'NONE', #53754, #50282, #25183, .T. ) ;
#42176=DIRECTION ( 'NONE',  ( 0.000000000000000000, 0.000000000000000000, -1.000000000000000000 ) ) ;
#42411=ORIENTED_EDGE ( 'NONE', *, *, #4432, .F. ) ;
#42425=VERTEX_POINT ( 'NONE', #18219 ) ;
#42443=ORIENTED_EDGE ( 'NONE', *, *, #68814, .F. ) ;
#42468=FACE_OUTER_BOUND ( 'NONE', #14762, .T. ) ;
#42830=VECTOR ( 'NONE', #38868, 1000.000000000000000 ) ;
#42839=CARTESIAN_POINT ( 'NONE',  ( 16.78635691501517613, 0.000000000000000000, -36.68900338898716740 ) ) ;
#42854=EDGE_LOOP ( 'NONE', ( #45965, #65055 ) ) ;
#42877=ADVANCED_FACE ( 'NONE', ( #11619 ), #33093, .T. ) ;
#42933=CARTESIAN_POINT ( 'NONE',  ( 16.78635691501517613, 6.000000000000000000, -9.435653166495500344 ) ) ;
#43016=CARTESIAN_POINT ( 'NONE',  ( 123.4242852856285566, 10.00000000000000000, -20.00000000000000000 ) ) ;
#43032=AXIS2_PLACEMENT_3D ( 'NONE', #44570, #39297, #27682 ) ;
#43052=VERTEX_POINT ( 'NONE', #22103 ) ;
#43202=CARTESIAN_POINT ( 'NONE',  ( 149.0250918491436778, 6.000000000000000000, -14.43565316649551811 ) ) ;
#43210=AXIS2_PLACEMENT_3D ( 'NONE', #58871, #43387, #839 ) ;
#43232=CARTESIAN_POINT ( 'NONE',  ( 149.0250918491436778, 6.000000000000000000, -9.435653166495526989 ) ) ;
#43328=CARTESIAN_POINT ( 'NONE',  ( 99.99999999999997158, 0.000000000000000000, -25.00000000000000000 ) ) ;
#43347=ORIENTED_EDGE ( 'NONE', *, *, #53818, .T. ) ;
#43387=DIRECTION ( 'NONE',  ( 0.5773502691896258421, 0.5773502691896258421, 0.5773502691896258421 ) ) ;
#43390=DIRECTION ( 'NONE',  ( 0.000000000000000000, -1.000000000000000000, 0.000000000000000000 ) ) ;
#43403=ADVANCED_FACE ( 'NONE', ( #4723 ), #62790, .T. ) ;
#43506=ADVANCED_FACE ( 'NONE', ( #27209 ), #21935, .T. ) ;
#43514=CARTESIAN_POINT ( 'NONE',  ( 16.78635691501517613, 6.000000000000000000, -9.435653166495500344 ) ) ;
#43527=CIRCLE ( 'NONE', #48043, 21.99999999999998579 ) ;
#43604=CARTESIAN_POINT ( 'NONE',  ( 183.2136430849847955, 6.000000000000000000, -41.68900338898720292 ) ) ;
#43671=ORIENTED_EDGE ( 'NONE', *, *, #39464, .T. ) ;
#43718=CARTESIAN_POINT ( 'NONE',  ( 149.0250918491436494, 0.000000000000000000, -41.68900338898718871 ) ) ;
#43757=CARTESIAN_POINT ( 'NONE',  ( 16.78635691501517613, 0.000000000000000000, -46.68900338898716029 ) ) ;
#43820=VECTOR ( 'NONE', #20526, 1000.000000000000114 ) ;
#43828=VERTEX_POINT ( 'NONE', #56915 ) ;
#43888=AXIS2_PLACEMENT_3D ( 'NONE', #52967, #63547, #4794 ) ;
#43942=LINE ( 'NONE', #36958, #7755 ) ;
#44010=LINE ( 'NONE', #10968, #66777 ) ;
#44092=ORIENTED_EDGE ( 'NONE', *, *, #51610, .T. ) ;
#44138=VERTEX_POINT ( 'NONE', #8183 ) ;
#44188=EDGE_CURVE ( 'NONE', #50693, #52936, #5316, .T. ) ;
#44240=EDGE_CURVE ( 'NONE', #32425, #41408, #11618, .T. ) ;
#44262=VERTEX_POINT ( 'NONE', #55229 ) ;
#44439=PLANE ( 'NONE',  #40756 ) ;
#44442=CARTESIAN_POINT ( 'NONE',  ( 121.4242852856285566, 0.000000000000000000, -30.00000000000000000 ) ) ;
#44469=ORIENTED_EDGE ( 'NONE', *, *, #57267, .F. ) ;
#44477=CARTESIAN_POINT ( 'NONE',  ( 76.57571471437145760, 0.000000000000000000, -20.00000000000000000 ) ) ;
#44481=LINE ( 'NONE', #169, #48437 ) ;
#44521=ADVANCED_FACE ( 'NONE', ( #60350 ), #16731, .T. ) ;
#44538=CARTESIAN_POINT ( 'NONE',  ( 1.500000000000013101, 4.499999999999984013, -3.000000000000029310 ) ) ;
#44542=ORIENTED_EDGE ( 'NONE', *, *, #36645, .F. ) ;
#44558=DIRECTION ( 'NONE',  ( 0.000000000000000000, 0.000000000000000000, 1.000000000000000000 ) ) ;
#44570=CARTESIAN_POINT ( 'NONE',  ( 183.2136430849848239, 6.000000000000000000, -9.435653166495541200 ) ) ;
#44595=ORIENTED_EDGE ( 'NONE', *, *, #28514, .T. ) ;
#44663=CARTESIAN_POINT ( 'NONE',  ( 0.000000000000000000, 6.000000000000000000, -3.000000000000030198 ) ) ;
#44692=DIRECTION ( 'NONE',  ( 0.000000000000000000, 0.000000000000000000, 1.000000000000000000 ) ) ;
#44698=CARTESIAN_POINT ( 'NONE',  ( 200.0000000000000000, 0.000000000000000000, -46.99999999999997158 ) ) ;
#44798=CARTESIAN_POINT ( 'NONE',  ( 3.000000000000003997, 1.500000000000015321, -48.49999999999998579 ) ) ;
#44847=VECTOR ( 'NONE', #25136, 1000.000000000000000 ) ;
#44858=ADVANCED_FACE ( 'NONE', ( #57506, #25510, #51542, #57164, #31129 ), #46591, .T. ) ;
#45110=AXIS2_PLACEMENT_3D ( 'NONE', #62615, #57681, #8806 ) ;
#45162=SURFACE_STYLE_FILL_AREA ( #23719 ) ;
#45177=LINE ( 'NONE', #1942, #69392 ) ;
#45267=VECTOR ( 'NONE', #12827, 1000.000000000000000 ) ;
#45276=EDGE_CURVE ( 'NONE', #5944, #43052, #8547, .T. ) ;
#45347=DIRECTION ( 'NONE',  ( 0.000000000000000000, -0.7071067811865475727, -0.7071067811865475727 ) ) ;
#45370=DIRECTION ( 'NONE',  ( -0.000000000000000000, -1.000000000000000000, -0.000000000000000000 ) ) ;
#45384=DIRECTION ( 'NONE',  ( 0.000000000000000000, 0.000000000000000000, 1.000000000000000000 ) ) ;
#45392=CARTESIAN_POINT ( 'NONE',  ( 3.000000000000028866, 0.000000000000000000, -3.000000000000030198 ) ) ;
#45536=ORIENTED_EDGE ( 'NONE', *, *, #14944, .F. ) ;
#45601=LINE ( 'NONE', #66392, #52433 ) ;
#45628=ORIENTED_EDGE ( 'NONE', *, *, #23537, .T. ) ;
#45812=EDGE_CURVE ( 'NONE', #30796, #32425, #22112, .T. ) ;
#45847=VERTEX_POINT ( 'NONE', #2065 ) ;
#45945=DIRECTION ( 'NONE',  ( 0.000000000000000000, 0.000000000000000000, 1.000000000000000000 ) ) ;
#45965=ORIENTED_EDGE ( 'NONE', *, *, #21999, .T. ) ;
#45978=EDGE_LOOP ( 'NONE', ( #5558, #10314 ) ) ;
#46017=DIRECTION ( 'NONE',  ( 0.000000000000000000, 0.000000000000000000, -1.000000000000000000 ) ) ;
#46060=DIRECTION ( 'NONE',  ( 0.000000000000000000, 0.000000000000000000, -1.000000000000000000 ) ) ;
#46212=ORIENTED_EDGE ( 'NONE', *, *, #14609, .T. ) ;
#46294=ORIENTED_EDGE ( 'NONE', *, *, #12875, .T. ) ;
#46401=CARTESIAN_POINT ( 'NONE',  ( 200.0000000000000000, 3.000000000000030198, -46.99999999999997158 ) ) ;
#46434=DIRECTION ( 'NONE',  ( 0.000000000000000000, 0.000000000000000000, 1.000000000000000000 ) ) ;
#46465=ORIENTED_EDGE ( 'NONE', *, *, #56947, .F. ) ;
#46510=EDGE_CURVE ( 'NONE', #5640, #65549, #39438, .T. ) ;
#46528=CARTESIAN_POINT ( 'NONE',  ( 149.0250918491436778, 0.000000000000000000, -9.435653166495526989 ) ) ;
#46591=PLANE ( 'NONE',  #30996 ) ;
#46707=FACE_OUTER_BOUND ( 'NONE', #14020, .T. ) ;
#46832=VERTEX_POINT ( 'NONE', #17550 ) ;
#46937=DIRECTION ( 'NONE',  ( 0.7071067811865475727, 0.000000000000000000, -0.7071067811865475727 ) ) ;
#47054=CARTESIAN_POINT ( 'NONE',  ( 149.0250918491436494, 6.000000000000000000, -41.68900338898718871 ) ) ;
#47055=CARTESIAN_POINT ( 'NONE',  ( 50.97490815085634352, 6.000000000000000000, -9.435653166495500344 ) ) ;
#47095=EDGE_CURVE ( 'NONE', #31811, #63882, #55805, .T. ) ;
#47136=LINE ( 'NONE', #53437, #7169 ) ;
#47145=ORIENTED_EDGE ( 'NONE', *, *, #38611, .F. ) ;
#47271=DIRECTION ( 'NONE',  ( 0.000000000000000000, 1.000000000000000000, -0.000000000000000000 ) ) ;
#47274=DIRECTION ( 'NONE',  ( 0.5773502691896258421, -0.5773502691896258421, -0.5773502691896258421 ) ) ;
#47285=ORIENTED_EDGE ( 'NONE', *, *, #51131, .F. ) ;
#47315=VECTOR ( 'NONE', #60638, 1000.000000000000000 ) ;
#47423=ORIENTED_EDGE ( 'NONE', *, *, #64707, .F. ) ;
#47427=CARTESIAN_POINT ( 'NONE',  ( 16.78635691501517613, 6.000000000000000000, -14.43565316649550034 ) ) ;
#47489=ORIENTED_EDGE ( 'NONE', *, *, #14226, .F. ) ;
#47501=DIRECTION ( 'NONE',  ( -0.000000000000000000, -1.000000000000000000, -0.000000000000000000 ) ) ;
#47502=EDGE_LOOP ( 'NONE', ( #30467, #60034, #69143 ) ) ;
#47521=ORIENTED_EDGE ( 'NONE', *, *, #31275, .T. ) ;
#47763=VECTOR ( 'NONE', #28951, 1000.000000000000000 ) ;
#47764=CARTESIAN_POINT ( 'NONE',  ( 78.57571471437144339, 6.000000000000000000, -20.00000000000000000 ) ) ;
#47785=ORIENTED_EDGE ( 'NONE', *, *, #6461, .F. ) ;
#47786=DIRECTION ( 'NONE',  ( -0.000000000000000000, -1.000000000000000000, -0.000000000000000000 ) ) ;
#47823=DIRECTION ( 'NONE',  ( 0.000000000000000000, 0.7071067811865474617, 0.7071067811865474617 ) ) ;
#47958=DIRECTION ( 'NONE',  ( -0.7071067811865475727, 0.000000000000000000, -0.7071067811865475727 ) ) ;
#47981=EDGE_LOOP ( 'NONE', ( #20230, #26866 ) ) ;
#48043=AXIS2_PLACEMENT_3D ( 'NONE', #40528, #29627, #12420 ) ;
#48227=AXIS2_PLACEMENT_3D ( 'NONE', #35348, #62066, #56807 ) ;
#48342=VECTOR ( 'NONE', #37557, 1000.000000000000000 ) ;
#48348=ORIENTED_EDGE ( 'NONE', *, *, #23531, .F. ) ;
#48362=DIRECTION ( 'NONE',  ( 0.000000000000000000, 0.000000000000000000, 1.000000000000000000 ) ) ;
#48437=VECTOR ( 'NONE', #54315, 1000.000000000000000 ) ;
#48452=ORIENTED_EDGE ( 'NONE', *, *, #68814, .T. ) ;
#48566=EDGE_LOOP ( 'NONE', ( #41574, #3357, #27792, #47489 ) ) ;
#48567=EDGE_CURVE ( 'NONE', #60670, #68142, #25673, .T. ) ;
#48668=ORIENTED_EDGE ( 'NONE', *, *, #56242, .T. ) ;
#48805=DIRECTION ( 'NONE',  ( 0.000000000000000000, 1.000000000000000000, 0.000000000000000000 ) ) ;
#48863=CARTESIAN_POINT ( 'NONE',  ( 50.97490815085634352, 0.000000000000000000, -9.435653166495500344 ) ) ;
#48927=DIRECTION ( 'NONE',  ( 0.000000000000000000, 0.000000000000000000, -1.000000000000000000 ) ) ;
#48930=ORIENTED_EDGE ( 'NONE', *, *, #3834, .T. ) ;
#49002=ORIENTED_EDGE ( 'NONE', *, *, #61614, .F. ) ;
#49081=VECTOR ( 'NONE', #13407, 1000.000000000000114 ) ;
#49085=EDGE_LOOP ( 'NONE', ( #9421, #55300, #22965, #36019 ) ) ;
#49253=LINE ( 'NONE', #44698, #20803 ) ;
#49282=ORIENTED_EDGE ( 'NONE', *, *, #64875, .F. ) ;
#49354=ORIENTED_EDGE ( 'NONE', *, *, #47095, .T. ) ;
#49364=ORIENTED_EDGE ( 'NONE', *, *, #62986, .F. ) ;
#49369=DIRECTION ( 'NONE',  ( 0.000000000000000000, -0.7071067811865474617, -0.7071067811865474617 ) ) ;
#49411=LINE ( 'NONE', #50127, #24467 ) ;
#49504=DIRECTION ( 'NONE',  ( 0.000000000000000000, 0.000000000000000000, 1.000000000000000000 ) ) ;
#49510=VECTOR ( 'NONE', #40604, 1000.000000000000000 ) ;
#49513=DIRECTION ( 'NONE',  ( -0.000000000000000000, -1.000000000000000000, -0.000000000000000000 ) ) ;
#49591=EDGE_LOOP ( 'NONE', ( #11533, #43347 ) ) ;
#49608=DIRECTION ( 'NONE',  ( 1.000000000000000000, 0.000000000000000000, -1.734723475976805517E-15 ) ) ;
#49648=CARTESIAN_POINT ( 'NONE',  ( 183.2136430849848239, 0.000000000000000000, -9.435653166495541200 ) ) ;
#49813=DIRECTION ( 'NONE',  ( -1.000000000000000000, 0.000000000000000000, 0.000000000000000000 ) ) ;
#50013=VECTOR ( 'NONE', #26434, 1000.000000000000000 ) ;
#50027=ORIENTED_EDGE ( 'NONE', *, *, #10389, .T. ) ;
#50075=CIRCLE ( 'NONE', #5123, 5.000000000000018652 ) ;
#50124=LINE ( 'NONE', #27963, #59384 ) ;
#50127=CARTESIAN_POINT ( 'NONE',  ( -2.609024107869115977E-14, 3.000000000000030198, -46.99999999999997158 ) ) ;
#50249=ORIENTED_EDGE ( 'NONE', *, *, #66286, .F. ) ;
#50271=ORIENTED_EDGE ( 'NONE', *, *, #67745, .F. ) ;
#50282=VERTEX_POINT ( 'NONE', #28673 ) ;
#50290=AXIS2_PLACEMENT_3D ( 'NONE', #42933, #64400, #54883 ) ;
#50300=EDGE_CURVE ( 'NONE', #5640, #42425, #49411, .T. ) ;
#50372=CARTESIAN_POINT ( 'NONE',  ( 99.99999999999997158, 6.000000000000000000, -25.00000000000000000 ) ) ;
#50411=DIRECTION ( 'NONE',  ( 1.000000000000000000, 0.000000000000000000, -0.000000000000000000 ) ) ;
#50492=VERTEX_POINT ( 'NONE', #62762 ) ;
#50505=EDGE_CURVE ( 'NONE', #11659, #6690, #29363, .T. ) ;
#50530=CARTESIAN_POINT ( 'NONE',  ( 0.000000000000000000, 0.000000000000000000, 0.000000000000000000 ) ) ;
#50593=CARTESIAN_POINT ( 'NONE',  ( 149.0250918491436778, 0.000000000000000000, -9.435653166495526989 ) ) ;
#50644=LINE ( 'NONE', #12321, #35332 ) ;
#50676=VERTEX_POINT ( 'NONE', #27356 ) ;
#50693=VERTEX_POINT ( 'NONE', #30496 ) ;
#50707=DIRECTION ( 'NONE',  ( -1.000000000000000000, 0.000000000000000000, -1.734723475976805517E-15 ) ) ;
#50744=EDGE_CURVE ( 'NONE', #69370, #30206, #21458, .T. ) ;
#50798=ORIENTED_EDGE ( 'NONE', *, *, #5461, .T. ) ;
#50837=ORIENTED_EDGE ( 'NONE', *, *, #30250, .F. ) ;
#50854=LINE ( 'NONE', #44538, #61794 ) ;
#50909=ORIENTED_EDGE ( 'NONE', *, *, #47095, .F. ) ;
#50980=ADVANCED_FACE ( 'NONE', ( #30414 ), #51866, .T. ) ;
#51016=DIRECTION ( 'NONE',  ( 1.000000000000000000, 0.000000000000000000, 0.000000000000000000 ) ) ;
#51052=ADVANCED_FACE ( 'NONE', ( #22274 ), #59891, .T. ) ;
#51060=LINE ( 'NONE', #23638, #28180 ) ;
#51131=EDGE_CURVE ( 'NONE', #41805, #10488, #39449, .T. ) ;
#51290=AXIS2_PLACEMENT_3D ( 'NONE', #22333, #33248, #4768 ) ;
#51385=CARTESIAN_POINT ( 'NONE',  ( 183.2136430849848239, 6.000000000000000000, -9.435653166495541200 ) ) ;
#51395=AXIS2_PLACEMENT_3D ( 'NONE', #11100, #65267, #48362 ) ;
#51453=VERTEX_POINT ( 'NONE', #16903 ) ;
#51456=FACE_OUTER_BOUND ( 'NONE', #48566, .T. ) ;
#51465=ORIENTED_EDGE ( 'NONE', *, *, #6648, .F. ) ;
#51542=FACE_BOUND ( 'NONE', #49591, .T. ) ;
#51543=EDGE_CURVE ( 'NONE', #41654, #62549, #5788, .T. ) ;
#51610=EDGE_CURVE ( 'NONE', #62549, #41654, #59657, .T. ) ;
#51618=EDGE_LOOP ( 'NONE', ( #33771, #26842, #7574, #6509 ) ) ;
#51732=ORIENTED_EDGE ( 'NONE', *, *, #5461, .F. ) ;
#51794=DIRECTION ( 'NONE',  ( 5.551115123125781716E-16, 0.000000000000000000, 1.000000000000000000 ) ) ;
#51866=PLANE ( 'NONE',  #55144 ) ;
#51907=( LENGTH_UNIT ( ) NAMED_UNIT ( * ) SI_UNIT ( .MILLI., .METRE. ) );
#51942=LINE ( 'NONE', #67788, #62290 ) ;
#52067=CARTESIAN_POINT ( 'NONE',  ( 16.78635691501517613, 0.000000000000000000, -9.435653166495500344 ) ) ;
#52139=AXIS2_PLACEMENT_3D ( 'NONE', #54204, #27488, #48927 ) ;
#52189=CIRCLE ( 'NONE', #27419, 5.000000000000018652 ) ;
#52333=CYLINDRICAL_SURFACE ( 'NONE', #52482, 4.999999999999997335 ) ;
#52337=AXIS2_PLACEMENT_3D ( 'NONE', #16350, #32877, #27593 ) ;
#52433=VECTOR ( 'NONE', #28736, 1000.000000000000000 ) ;
#52434=ORIENTED_EDGE ( 'NONE', *, *, #60180, .F. ) ;
#52482=AXIS2_PLACEMENT_3D ( 'NONE', #47055, #20319, #63238 ) ;
#52495=FACE_OUTER_BOUND ( 'NONE', #29244, .T. ) ;
#52588=CARTESIAN_POINT ( 'NONE',  ( 76.57571471437145760, 6.000000000000000000, -20.00000000000000000 ) ) ;
#52597=DIRECTION ( 'NONE',  ( 0.000000000000000000, 1.000000000000000000, 0.000000000000000000 ) ) ;
#52716=EDGE_LOOP ( 'NONE', ( #2621, #9400, #51465, #18642 ) ) ;
#52727=VECTOR ( 'NONE', #49513, 1000.000000000000000 ) ;
#52873=LINE ( 'NONE', #14571, #64544 ) ;
#52915=ORIENTED_EDGE ( 'NONE', *, *, #17367, .F. ) ;
#52936=VERTEX_POINT ( 'NONE', #42839 ) ;
#52947=CARTESIAN_POINT ( 'NONE',  ( 121.4242852856285140, 6.000000000000000000, -30.00000000000000355 ) ) ;
#52967=CARTESIAN_POINT ( 'NONE',  ( 149.0250918491436494, 0.000000000000000000, -41.68900338898718871 ) ) ;
#53121=ORIENTED_EDGE ( 'NONE', *, *, #53818, .F. ) ;
#53156=VECTOR ( 'NONE', #28290, 1000.000000000000000 ) ;
#53323=AXIS2_PLACEMENT_3D ( 'NONE', #62116, #52597, #45945 ) ;
#53397=CARTESIAN_POINT ( 'NONE',  ( 16.78635691501517613, 6.000000000000000000, -9.435653166495500344 ) ) ;
#53437=CARTESIAN_POINT ( 'NONE',  ( 3.000000000000004441, 2.999999999999969802, -50.00000000000000000 ) ) ;
#53483=EDGE_LOOP ( 'NONE', ( #19751, #11329, #7145, #63187, #25707, #33747, #32231, #6538 ) ) ;
#53590=VERTEX_POINT ( 'NONE', #5099 ) ;
#53733=EDGE_LOOP ( 'NONE', ( #50837, #67716 ) ) ;
#53754=VERTEX_POINT ( 'NONE', #69383 ) ;
#53818=EDGE_CURVE ( 'NONE', #8968, #35032, #7108, .T. ) ;
#53825=CARTESIAN_POINT ( 'NONE',  ( 183.2136430849847955, 6.000000000000000000, -46.68900338898722424 ) ) ;
#53877=DIRECTION ( 'NONE',  ( 0.000000000000000000, 1.000000000000000000, -0.000000000000000000 ) ) ;
#53942=ORIENTED_EDGE ( 'NONE', *, *, #12785, .T. ) ;
#53949=EDGE_LOOP ( 'NONE', ( #25704, #67807, #31872, #4278 ) ) ;
#53972=DIRECTION ( 'NONE',  ( 0.000000000000000000, 1.000000000000000000, 0.000000000000000000 ) ) ;
#53978=CARTESIAN_POINT ( 'NONE',  ( 196.9999999999999716, 0.000000000000000000, -46.99999999999997158 ) ) ;
#53980=ORIENTED_EDGE ( 'NONE', *, *, #12785, .F. ) ;
#54005=FACE_BOUND ( 'NONE', #12940, .T. ) ;
#54016=EDGE_CURVE ( 'NONE', #6148, #31811, #29595, .T. ) ;
#54038=ORIENTED_EDGE ( 'NONE', *, *, #24486, .T. ) ;
#54071=ORIENTED_EDGE ( 'NONE', *, *, #31011, .F. ) ;
#54204=CARTESIAN_POINT ( 'NONE',  ( 149.0250918491436778, 6.000000000000000000, -9.435653166495526989 ) ) ;
#54257=DIRECTION ( 'NONE',  ( 0.000000000000000000, 0.000000000000000000, -1.000000000000000000 ) ) ;
#54270=ADVANCED_FACE ( 'NONE', ( #12214 ), #33333, .F. ) ;
#54294=FACE_OUTER_BOUND ( 'NONE', #57065, .T. ) ;
#54315=DIRECTION ( 'NONE',  ( 0.000000000000000000, 0.000000000000000000, -1.000000000000000000 ) ) ;
#54388=DIRECTION ( 'NONE',  ( 0.000000000000000000, 0.000000000000000000, -1.000000000000000000 ) ) ;
#54409=FACE_OUTER_BOUND ( 'NONE', #49085, .T. ) ;
#54419=AXIS2_PLACEMENT_3D ( 'NONE', #50372, #38775, #7104 ) ;
#54497=ORIENTED_EDGE ( 'NONE', *, *, #38611, .T. ) ;
#54696=DIRECTION ( 'NONE',  ( -1.000000000000000000, 0.000000000000000000, 0.000000000000000000 ) ) ;
#54723=ORIENTED_EDGE ( 'NONE', *, *, #50744, .T. ) ;
#54869=EDGE_CURVE ( 'NONE', #51453, #17220, #19504, .T. ) ;
#54883=DIRECTION ( 'NONE',  ( 0.000000000000000000, 0.000000000000000000, 1.000000000000000000 ) ) ;
#54886=DIRECTION ( 'NONE',  ( 1.000000000000000000, 0.000000000000000000, 0.000000000000000000 ) ) ;
#54978=DIRECTION ( 'NONE',  ( 0.000000000000000000, 0.000000000000000000, -1.000000000000000000 ) ) ;
#55017=CARTESIAN_POINT ( 'NONE',  ( 183.2136430849847955, 0.000000000000000000, -41.68900338898720292 ) ) ;
#55026=DIRECTION ( 'NONE',  ( -0.000000000000000000, -1.000000000000000000, -0.000000000000000000 ) ) ;
#55038=DIRECTION ( 'NONE',  ( -0.7071067811865475727, -0.7071067811865475727, -0.000000000000000000 ) ) ;
#55144=AXIS2_PLACEMENT_3D ( 'NONE', #4029, #25501, #46937 ) ;
#55171=DIRECTION ( 'NONE',  ( 0.000000000000000000, 0.000000000000000000, 1.000000000000000000 ) ) ;
#55229=CARTESIAN_POINT ( 'NONE',  ( 196.9999999999999716, 3.000000000000030198, -50.00000000000000000 ) ) ;
#55300=ORIENTED_EDGE ( 'NONE', *, *, #26790, .T. ) ;
#55307=ORIENTED_EDGE ( 'NONE', *, *, #26790, .F. ) ;
#55311=CARTESIAN_POINT ( 'NONE',  ( 99.99999999999997158, 6.000000000000000000, -46.99999999999997158 ) ) ;
#55337=FACE_BOUND ( 'NONE', #4785, .T. ) ;
#55339=ORIENTED_EDGE ( 'NONE', *, *, #62746, .F. ) ;
#55347=CARTESIAN_POINT ( 'NONE',  ( 183.2136430849847955, 0.000000000000000000, -41.68900338898720292 ) ) ;
#55374=LINE ( 'NONE', #7198, #27114 ) ;
#55500=DIRECTION ( 'NONE',  ( -1.000000000000000000, 0.000000000000000000, 0.000000000000000000 ) ) ;
#55558=DIRECTION ( 'NONE',  ( 0.000000000000000000, 1.000000000000000000, 0.000000000000000000 ) ) ;
#55582=CARTESIAN_POINT ( 'NONE',  ( 196.9999999999999716, 0.000000000000000000, 0.000000000000000000 ) ) ;
#55627=DIRECTION ( 'NONE',  ( 0.000000000000000000, -0.7071067811865474617, -0.7071067811865474617 ) ) ;
#55695=ORIENTED_EDGE ( 'NONE', *, *, #44240, .T. ) ;
#55707=ORIENTED_EDGE ( 'NONE', *, *, #41782, .T. ) ;
#55711=LINE ( 'NONE', #11389, #47315 ) ;
#55805=LINE ( 'NONE', #17825, #57005 ) ;
#55821=ADVANCED_FACE ( 'NONE', ( #23319 ), #28582, .T. ) ;
#55939=EDGE_LOOP ( 'NONE', ( #54723, #59790 ) ) ;
#55946=DIRECTION ( 'NONE',  ( -0.5773502691896255090, 0.5773502691896258421, 0.5773502691896258421 ) ) ;
#55980=ORIENTED_EDGE ( 'NONE', *, *, #46510, .T. ) ;
#56019=ORIENTED_EDGE ( 'NONE', *, *, #2481, .T. ) ;
#56034=ORIENTED_EDGE ( 'NONE', *, *, #67745, .T. ) ;
#56047=VERTEX_POINT ( 'NONE', #39366 ) ;
#56158=ORIENTED_EDGE ( 'NONE', *, *, #57029, .F. ) ;
#56179=DIRECTION ( 'NONE',  ( -1.000000000000000000, -0.000000000000000000, -0.000000000000000000 ) ) ;
#56215=ORIENTED_EDGE ( 'NONE', *, *, #67271, .T. ) ;
#56220=CARTESIAN_POINT ( 'NONE',  ( 50.97490815085634352, 0.000000000000000000, -14.43565316649549679 ) ) ;
#56242=EDGE_CURVE ( 'NONE', #6148, #21697, #51942, .T. ) ;
#56263=AXIS2_PLACEMENT_3D ( 'NONE', #43016, #54257, #22979 ) ;
#56404=UNCERTAINTY_MEASURE_WITH_UNIT (LENGTH_MEASURE( 1.000000000000000082E-05 ), #66641, 'distance_accuracy_value', 'NONE');
#56449=CARTESIAN_POINT ( 'NONE',  ( 3.000000000000028866, 2.999999999999969802, 0.000000000000000000 ) ) ;
#56504=CARTESIAN_POINT ( 'NONE',  ( 149.0250918491436494, 6.000000000000000000, -36.68900338898720292 ) ) ;
#56591=DIRECTION ( 'NONE',  ( 0.000000000000000000, 0.000000000000000000, 1.000000000000000000 ) ) ;
#56600=VECTOR ( 'NONE', #26403, 1000.000000000000000 ) ;
#56632=DIRECTION ( 'NONE',  ( 0.000000000000000000, 1.000000000000000000, -0.000000000000000000 ) ) ;
#56680=CARTESIAN_POINT ( 'NONE',  ( 183.2136430849847955, 0.000000000000000000, -46.68900338898722424 ) ) ;
#56807=DIRECTION ( 'NONE',  ( 0.000000000000000000, 0.000000000000000000, 1.000000000000000000 ) ) ;
#56817=VECTOR ( 'NONE', #10216, 1000.000000000000114 ) ;
#56915=CARTESIAN_POINT ( 'NONE',  ( 50.97490815085634352, 6.000000000000000000, -14.43565316649549679 ) ) ;
#56932=CARTESIAN_POINT ( 'NONE',  ( 183.2136430849848239, 6.000000000000000000, -9.435653166495541200 ) ) ;
#56936=CYLINDRICAL_SURFACE ( 'NONE', #18503, 21.99999999999998579 ) ;
#56947=EDGE_CURVE ( 'NONE', #41805, #53590, #14410, .T. ) ;
#56977=VERTEX_POINT ( 'NONE', #46401 ) ;
#56981=ORIENTED_EDGE ( 'NONE', *, *, #5076, .T. ) ;
#57005=VECTOR ( 'NONE', #49813, 1000.000000000000000 ) ;
#57029=EDGE_CURVE ( 'NONE', #35032, #8968, #17431, .T. ) ;
#57054=ORIENTED_EDGE ( 'NONE', *, *, #66286, .T. ) ;
#57059=VECTOR ( 'NONE', #29098, 1000.000000000000000 ) ;
#57065=EDGE_LOOP ( 'NONE', ( #35447, #4168, #40702 ) ) ;
#57107=CIRCLE ( 'NONE', #24533, 4.999999999999996447 ) ;
#57111=CIRCLE ( 'NONE', #33519, 4.999999999999990230 ) ;
#57154=VECTOR ( 'NONE', #978, 1000.000000000000000 ) ;
#57157=ORIENTED_EDGE ( 'NONE', *, *, #6323, .T. ) ;
#57164=FACE_BOUND ( 'NONE', #55939, .T. ) ;
#57168=CARTESIAN_POINT ( 'NONE',  ( -2.609024107869115977E-14, 3.000000000000030198, -46.99999999999997158 ) ) ;
#57253=VECTOR ( 'NONE', #38511, 1000.000000000000000 ) ;
#57257=CARTESIAN_POINT ( 'NONE',  ( 16.78635691501517613, 6.000000000000000000, -41.68900338898716740 ) ) ;
#57261=ADVANCED_FACE ( 'NONE', ( #25584 ), #67795, .F. ) ;
#57267=EDGE_CURVE ( 'NONE', #67476, #44138, #67451, .T. ) ;
#57279=CARTESIAN_POINT ( 'NONE',  ( 99.99999999999997158, 6.000000000000000000, -25.00000000000000000 ) ) ;
#57295=ORIENTED_EDGE ( 'NONE', *, *, #54869, .T. ) ;
#57382=DIRECTION ( 'NONE',  ( -0.000000000000000000, -1.000000000000000000, -0.000000000000000000 ) ) ;
#57506=FACE_BOUND ( 'NONE', #34596, .T. ) ;
#57558=ORIENTED_EDGE ( 'NONE', *, *, #32326, .T. ) ;
#57674=AXIS2_PLACEMENT_3D ( 'NONE', #66429, #47271, #68723 ) ;
#57681=DIRECTION ( 'NONE',  ( 0.000000000000000000, 1.000000000000000000, -0.000000000000000000 ) ) ;
#57717=ORIENTED_EDGE ( 'NONE', *, *, #14777, .F. ) ;
#57743=ADVANCED_FACE ( 'NONE', ( #5740 ), #25842, .T. ) ;
#57760=FACE_OUTER_BOUND ( 'NONE', #60685, .T. ) ;
#57817=AXIS2_PLACEMENT_3D ( 'NONE', #69536, #37533, #60024 ) ;
#57827=EDGE_CURVE ( 'NONE', #40256, #62711, #38813, .T. ) ;
#57854=FACE_BOUND ( 'NONE', #61950, .T. ) ;
#57924=CARTESIAN_POINT ( 'NONE',  ( 0.000000000000000000, 2.999999999999969802, 0.000000000000000000 ) ) ;
#57951=CARTESIAN_POINT ( 'NONE',  ( 183.2136430849848239, 6.000000000000000000, -14.43565316649556074 ) ) ;
#58102=DIRECTION ( 'NONE',  ( 0.000000000000000000, 0.000000000000000000, -1.000000000000000000 ) ) ;
#58106=CARTESIAN_POINT ( 'NONE',  ( 50.97490815085634352, 6.000000000000000000, -4.435653166495503896 ) ) ;
#58121=CARTESIAN_POINT ( 'NONE',  ( 149.0250918491436494, 6.000000000000000000, -46.68900338898718161 ) ) ;
#58198=AXIS2_PLACEMENT_3D ( 'NONE', #60837, #55558, #12658 ) ;
#58199=DIRECTION ( 'NONE',  ( 0.000000000000000000, 0.000000000000000000, -1.000000000000000000 ) ) ;
#58221=( NAMED_UNIT ( * ) SI_UNIT ( $, .STERADIAN. ) SOLID_ANGLE_UNIT ( ) );
#58255=ORIENTED_EDGE ( 'NONE', *, *, #51131, .T. ) ;
#58287=CARTESIAN_POINT ( 'NONE',  ( 121.4242852856285566, 6.000000000000000000, -30.00000000000000000 ) ) ;
#58395=DIRECTION ( 'NONE',  ( -0.000000000000000000, -1.000000000000000000, -0.000000000000000000 ) ) ;
#58467=AXIS2_PLACEMENT_3D ( 'NONE', #65047, #65399, #11559 ) ;
#58492=CARTESIAN_POINT ( 'NONE',  ( 183.2136430849847955, 0.000000000000000000, -36.68900338898718871 ) ) ;
#58606=FACE_BOUND ( 'NONE', #53733, .T. ) ;
#58653=DIRECTION ( 'NONE',  ( 0.000000000000000000, 0.000000000000000000, 1.000000000000000000 ) ) ;
#58830=DIRECTION ( 'NONE',  ( 0.000000000000000000, 1.000000000000000000, 0.000000000000000000 ) ) ;
#58869=LINE ( 'NONE', #21584, #9674 ) ;
#58871=CARTESIAN_POINT ( 'NONE',  ( 196.9999999999999716, 2.999999999999969802, 0.000000000000000000 ) ) ;
#58956=FACE_BOUND ( 'NONE', #47981, .T. ) ;
#59017=DIRECTION ( 'NONE',  ( 1.000000000000000000, 0.000000000000000000, 0.000000000000000000 ) ) ;
#59073=CARTESIAN_POINT ( 'NONE',  ( 16.78635691501517613, 0.000000000000000000, -14.43565316649550034 ) ) ;
#59089=ORIENTED_EDGE ( 'NONE', *, *, #27062, .F. ) ;
#59188=CARTESIAN_POINT ( 'NONE',  ( 200.0000000000000000, 3.000000000000030198, -3.000000000000030198 ) ) ;
#59195=ORIENTED_EDGE ( 'NONE', *, *, #3493, .F. ) ;
#59247=AXIS2_PLACEMENT_3D ( 'NONE', #33456, #1431, #45384 ) ;
#59261=DIRECTION ( 'NONE',  ( -5.551115123125781716E-16, 0.000000000000000000, -1.000000000000000000 ) ) ;
#59362=CARTESIAN_POINT ( 'NONE',  ( 0.000000000000000000, 6.000000000000000000, -3.000000000000030198 ) ) ;
#59384=VECTOR ( 'NONE', #28311, 1000.000000000000000 ) ;
#59398=ORIENTED_EDGE ( 'NONE', *, *, #62580, .F. ) ;
#59546=EDGE_LOOP ( 'NONE', ( #21396, #38680, #49354, #1772, #29487, #64862, #55307, #11232 ) ) ;
#59567=LINE ( 'NONE', #60977, #22515 ) ;
#59590=CARTESIAN_POINT ( 'NONE',  ( 183.2136430849848239, 6.000000000000000000, -4.435653166495524324 ) ) ;
#59608=VERTEX_POINT ( 'NONE', #29936 ) ;
#59657=CIRCLE ( 'NONE', #45110, 4.999999999999990230 ) ;
#59748=CIRCLE ( 'NONE', #30561, 4.999999999999997335 ) ;
#59790=ORIENTED_EDGE ( 'NONE', *, *, #63693, .T. ) ;
#59840=EDGE_CURVE ( 'NONE', #10488, #41805, #63534, .T. ) ;
#59891=PLANE ( 'NONE',  #56263 ) ;
#59901=CIRCLE ( 'NONE', #38583, 5.000000000000000888 ) ;
#60024=DIRECTION ( 'NONE',  ( 0.000000000000000000, 0.000000000000000000, -1.000000000000000000 ) ) ;
#60034=ORIENTED_EDGE ( 'NONE', *, *, #61614, .T. ) ;
#60123=EDGE_LOOP ( 'NONE', ( #21155, #63542, #12287 ) ) ;
#60180=EDGE_CURVE ( 'NONE', #12136, #7089, #20249, .T. ) ;
#60205=VECTOR ( 'NONE', #3955, 1000.000000000000000 ) ;
#60338=EDGE_CURVE ( 'NONE', #50693, #30445, #10749, .T. ) ;
#60350=FACE_OUTER_BOUND ( 'NONE', #69479, .T. ) ;
#60356=DIRECTION ( 'NONE',  ( 0.000000000000000000, 0.000000000000000000, -1.000000000000000000 ) ) ;
#60379=DIRECTION ( 'NONE',  ( 0.000000000000000000, 1.000000000000000000, 0.000000000000000000 ) ) ;
#60412=ORIENTED_EDGE ( 'NONE', *, *, #31275, .F. ) ;
#60424=AXIS2_PLACEMENT_3D ( 'NONE', #62350, #30342, #51794 ) ;
#60550=DIRECTION ( 'NONE',  ( 0.000000000000000000, 0.7071067811865474617, -0.7071067811865474617 ) ) ;
#60638=DIRECTION ( 'NONE',  ( 1.000000000000000000, 0.000000000000000000, 0.000000000000000000 ) ) ;
#60662=CARTESIAN_POINT ( 'NONE',  ( 3.000000000000002665, 0.000000000000000000, -50.00000000000000000 ) ) ;
#60670=VERTEX_POINT ( 'NONE', #20506 ) ;
#60685=EDGE_LOOP ( 'NONE', ( #42411, #12165, #47521, #47423 ) ) ;
#60770=CARTESIAN_POINT ( 'NONE',  ( 50.97490815085634352, 6.000000000000000000, -9.435653166495500344 ) ) ;
#60797=CARTESIAN_POINT ( 'NONE',  ( 50.97490815085634352, 0.000000000000000000, -41.68900338898716740 ) ) ;
#60837=CARTESIAN_POINT ( 'NONE',  ( 99.99999999999997158, 6.000000000000000000, -25.00000000000000000 ) ) ;
#60893=CARTESIAN_POINT ( 'NONE',  ( 183.2136430849848239, 0.000000000000000000, -4.435653166495524324 ) ) ;
#60977=CARTESIAN_POINT ( 'NONE',  ( 0.000000000000000000, 6.000000000000000000, -46.99999999999997158 ) ) ;
#61105=ADVANCED_FACE ( 'NONE', ( #26573 ), #175, .T. ) ;
#61193=CARTESIAN_POINT ( 'NONE',  ( 76.57571471437145760, 10.00000000000000000, -20.00000000000000000 ) ) ;
#61221=CARTESIAN_POINT ( 'NONE',  ( 149.0250918491436494, 6.000000000000000000, -41.68900338898718871 ) ) ;
#61226=VECTOR ( 'NONE', #49608, 1000.000000000000000 ) ;
#61265=DIRECTION ( 'NONE',  ( -0.7071067811865474617, 0.000000000000000000, 0.7071067811865475727 ) ) ;
#61381=ORIENTED_EDGE ( 'NONE', *, *, #69057, .T. ) ;
#61424=CARTESIAN_POINT ( 'NONE',  ( 121.4242852856285140, 6.000000000000000000, -20.00000000000000000 ) ) ;
#61432=ORIENTED_EDGE ( 'NONE', *, *, #12862, .T. ) ;
#61614=EDGE_CURVE ( 'NONE', #64271, #67476, #28931, .T. ) ;
#61676=ORIENTED_EDGE ( 'NONE', *, *, #6986, .F. ) ;
#61689=( NAMED_UNIT ( * ) PLANE_ANGLE_UNIT ( ) SI_UNIT ( $, .RADIAN. ) );
#61691=CARTESIAN_POINT ( 'NONE',  ( -1.665334536937750193E-15, 2.999999999999969358, -3.000000000000028422 ) ) ;
#61794=VECTOR ( 'NONE', #18853, 1000.000000000000114 ) ;
#61839=AXIS2_PLACEMENT_3D ( 'NONE', #39708, #67157, #28453 ) ;
#61913=ORIENTED_EDGE ( 'NONE', *, *, #37079, .F. ) ;
#61950=EDGE_LOOP ( 'NONE', ( #59398, #15557 ) ) ;
#62000=EDGE_LOOP ( 'NONE', ( #1616, #34574, #52434, #28256 ) ) ;
#62024=UNCERTAINTY_MEASURE_WITH_UNIT (LENGTH_MEASURE( 1.000000000000000082E-05 ), #51907, 'distance_accuracy_value', 'NONE');
#62066=DIRECTION ( 'NONE',  ( 0.000000000000000000, 1.000000000000000000, 0.000000000000000000 ) ) ;
#62116=CARTESIAN_POINT ( 'NONE',  ( 16.78635691501517613, 0.000000000000000000, -41.68900338898716740 ) ) ;
#62162=COLOUR_RGB ( '',0.7921568627450980005, 0.8196078431372548767, 0.9333333333333333481 ) ;
#62212=CARTESIAN_POINT ( 'NONE',  ( 99.99999999999997158, 0.000000000000000000, -46.99999999999997158 ) ) ;
#62290=VECTOR ( 'NONE', #56179, 1000.000000000000000 ) ;
#62350=CARTESIAN_POINT ( 'NONE',  ( 3.000000000000030198, 6.000000000000000000, -1.665334536937751377E-15 ) ) ;
#62549=VERTEX_POINT ( 'NONE', #32563 ) ;
#62580=EDGE_CURVE ( 'NONE', #43828, #5944, #65967, .T. ) ;
#62585=ORIENTED_EDGE ( 'NONE', *, *, #64314, .F. ) ;
#62598=ORIENTED_EDGE ( 'NONE', *, *, #41782, .F. ) ;
#62615=CARTESIAN_POINT ( 'NONE',  ( 149.0250918491436494, 6.000000000000000000, -41.68900338898718871 ) ) ;
#62654=CARTESIAN_POINT ( 'NONE',  ( 16.78635691501517613, 6.000000000000000000, -46.68900338898716029 ) ) ;
#62685=CARTESIAN_POINT ( 'NONE',  ( 50.97490815085634352, 6.000000000000000000, -41.68900338898716740 ) ) ;
#62711=VERTEX_POINT ( 'NONE', #18476 ) ;
#62746=EDGE_CURVE ( 'NONE', #44262, #1254, #40966, .T. ) ;
#62760=CARTESIAN_POINT ( 'NONE',  ( 0.000000000000000000, 6.000000000000000000, -20.00000000000000000 ) ) ;
#62762=CARTESIAN_POINT ( 'NONE',  ( 200.0000000000000000, 3.000000000000030198, -3.000000000000030198 ) ) ;
#62790=PLANE ( 'NONE',  #65698 ) ;
#62986=EDGE_CURVE ( 'NONE', #27414, #30796, #43527, .T. ) ;
#63181=VERTEX_POINT ( 'NONE', #53825 ) ;
#63187=ORIENTED_EDGE ( 'NONE', *, *, #57827, .T. ) ;
#63238=DIRECTION ( 'NONE',  ( 0.000000000000000000, 0.000000000000000000, -1.000000000000000000 ) ) ;
#63392=VECTOR ( 'NONE', #2169, 1000.000000000000114 ) ;
#63447=VECTOR ( 'NONE', #8629, 1000.000000000000114 ) ;
#63488=FACE_BOUND ( 'NONE', #29028, .T. ) ;
#63534=CIRCLE ( 'NONE', #11800, 4.999999999999990230 ) ;
#63542=ORIENTED_EDGE ( 'NONE', *, *, #46510, .F. ) ;
#63547=DIRECTION ( 'NONE',  ( 0.000000000000000000, 1.000000000000000000, -0.000000000000000000 ) ) ;
#63586=CIRCLE ( 'NONE', #15281, 4.999999999999997335 ) ;
#63693=EDGE_CURVE ( 'NONE', #30206, #69370, #57111, .T. ) ;
#63721=ADVANCED_FACE ( 'NONE', ( #19427 ), #8544, .F. ) ;
#63827=DIRECTION ( 'NONE',  ( 0.000000000000000000, 1.000000000000000000, -0.000000000000000000 ) ) ;
#63839=ORIENTED_EDGE ( 'NONE', *, *, #1260, .F. ) ;
#63882=VERTEX_POINT ( 'NONE', #45392 ) ;
#63996=ORIENTED_EDGE ( 'NONE', *, *, #68607, .F. ) ;
#64021=EDGE_LOOP ( 'NONE', ( #5637, #29908, #49364, #35167 ) ) ;
#64063=AXIS2_PLACEMENT_3D ( 'NONE', #897, #34665, #54696 ) ;
#64100=VECTOR ( 'NONE', #27398, 1000.000000000000000 ) ;
#64125=ORIENTED_EDGE ( 'NONE', *, *, #62746, .T. ) ;
#64271=VERTEX_POINT ( 'NONE', #33066 ) ;
#64314=EDGE_CURVE ( 'NONE', #40256, #34571, #43942, .T. ) ;
#64383=AXIS2_PLACEMENT_3D ( 'NONE', #43328, #16605, #56591 ) ;
#64400=DIRECTION ( 'NONE',  ( 0.000000000000000000, 1.000000000000000000, 0.000000000000000000 ) ) ;
#64544=VECTOR ( 'NONE', #20524, 1000.000000000000000 ) ;
#64569=DIRECTION ( 'NONE',  ( 0.000000000000000000, 0.000000000000000000, 1.000000000000000000 ) ) ;
#64574=AXIS2_PLACEMENT_3D ( 'NONE', #6355, #55946, #24292 ) ;
#64706=DIRECTION ( 'NONE',  ( 0.000000000000000000, 0.000000000000000000, -1.000000000000000000 ) ) ;
#64707=EDGE_CURVE ( 'NONE', #46832, #50676, #65082, .T. ) ;
#64797=PRODUCT_DEFINITION_CONTEXT ( 'detailed design', #435, 'design' ) ;
#64862=ORIENTED_EDGE ( 'NONE', *, *, #33445, .T. ) ;
#64865=CYLINDRICAL_SURFACE ( 'NONE', #26734, 4.999999999999997335 ) ;
#64875=EDGE_CURVE ( 'NONE', #27414, #22171, #533, .T. ) ;
#64901=EDGE_CURVE ( 'NONE', #43828, #28243, #1231, .T. ) ;
#64998=LINE ( 'NONE', #11505, #57154 ) ;
#65047=CARTESIAN_POINT ( 'NONE',  ( 99.99999999999997158, 6.000000000000000000, -25.00000000000000000 ) ) ;
#65050=CARTESIAN_POINT ( 'NONE',  ( 200.0000000000000000, 3.000000000000030198, -46.99999999999997158 ) ) ;
#65055=ORIENTED_EDGE ( 'NONE', *, *, #64707, .T. ) ;
#65057=DIRECTION ( 'NONE',  ( 0.000000000000000000, 1.000000000000000000, -0.000000000000000000 ) ) ;
#65082=CIRCLE ( 'NONE', #26914, 4.999999999999997335 ) ;
#65267=DIRECTION ( 'NONE',  ( 0.000000000000000000, 1.000000000000000000, 0.000000000000000000 ) ) ;
#65378=ORIENTED_EDGE ( 'NONE', *, *, #34300, .F. ) ;
#65399=DIRECTION ( 'NONE',  ( 0.000000000000000000, 1.000000000000000000, 0.000000000000000000 ) ) ;
#65462=ORIENTED_EDGE ( 'NONE', *, *, #44188, .F. ) ;
#65545=DIRECTION ( 'NONE',  ( 1.000000000000000000, 0.000000000000000000, -1.734723475976805517E-15 ) ) ;
#65549=VERTEX_POINT ( 'NONE', #27701 ) ;
#65576=ORIENTED_EDGE ( 'NONE', *, *, #18428, .T. ) ;
#65613=EDGE_LOOP ( 'NONE', ( #3530, #56215, #37125, #47145 ) ) ;
#65698=AXIS2_PLACEMENT_3D ( 'NONE', #57168, #9319, #41337 ) ;
#65710=ORIENTED_EDGE ( 'NONE', *, *, #37079, .T. ) ;
#65724=ORIENTED_EDGE ( 'NONE', *, *, #8093, .F. ) ;
#65783=DIRECTION ( 'NONE',  ( 0.7071067811865474617, -0.7071067811865474617, -3.951729029292866070E-16 ) ) ;
#65785=DIRECTION ( 'NONE',  ( -0.000000000000000000, -1.000000000000000000, -0.000000000000000000 ) ) ;
#65801=AXIS2_PLACEMENT_3D ( 'NONE', #26010, #68568, #33632 ) ;
#65837=DIRECTION ( 'NONE',  ( 0.000000000000000000, 0.000000000000000000, -1.000000000000000000 ) ) ;
#65905=CARTESIAN_POINT ( 'NONE',  ( 196.9999999999999716, 2.999999999999969802, 0.000000000000000000 ) ) ;
#65967=CIRCLE ( 'NONE', #51395, 4.999999999999996447 ) ;
#66011=ADVANCED_FACE ( 'NONE', ( #12152 ), #29368, .F. ) ;
#66032=DIRECTION ( 'NONE',  ( -0.000000000000000000, -1.000000000000000000, -0.000000000000000000 ) ) ;
#66089=EDGE_LOOP ( 'NONE', ( #54038, #44595, #45536, #11068, #10452, #57295 ) ) ;
#66145=LINE ( 'NONE', #61193, #40234 ) ;
#66252=ORIENTED_EDGE ( 'NONE', *, *, #14777, .T. ) ;
#66286=EDGE_CURVE ( 'NONE', #41408, #50492, #68717, .T. ) ;
#66316=LINE ( 'NONE', #29348, #69089 ) ;
#66385=VECTOR ( 'NONE', #65783, 1000.000000000000114 ) ;
#66392=CARTESIAN_POINT ( 'NONE',  ( 76.57571471437145760, 6.000000000000000000, 0.000000000000000000 ) ) ;
#66403=VERTEX_POINT ( 'NONE', #55311 ) ;
#66428=AXIS2_PLACEMENT_3D ( 'NONE', #17662, #18349, #61265 ) ;
#66429=CARTESIAN_POINT ( 'NONE',  ( 183.2136430849847955, 6.000000000000000000, -41.68900338898720292 ) ) ;
#66494=LINE ( 'NONE', #28848, #40851 ) ;
#66560=PLANE ( 'NONE',  #66428 ) ;
#66599=CARTESIAN_POINT ( 'NONE',  ( 78.57571471437144339, 6.000000000000000000, -30.00000000000000355 ) ) ;
#66632=VECTOR ( 'NONE', #21938, 1000.000000000000114 ) ;
#66641=( LENGTH_UNIT ( ) NAMED_UNIT ( * ) SI_UNIT ( .MILLI., .METRE. ) );
#66730=AXIS2_PLACEMENT_3D ( 'NONE', #38932, #60379, #12194 ) ;
#66777=VECTOR ( 'NONE', #60550, 1000.000000000000114 ) ;
#66832=AXIS2_PLACEMENT_3D ( 'NONE', #50530, #44558, #8319 ) ;
#66883=DIRECTION ( 'NONE',  ( -0.000000000000000000, -1.000000000000000000, -0.000000000000000000 ) ) ;
#66913=VECTOR ( 'NONE', #44692, 1000.000000000000000 ) ;
#66996=FILL_AREA_STYLE_COLOUR ( '', #62162 ) ;
#67109=EDGE_LOOP ( 'NONE', ( #31573, #47285 ) ) ;
#67113=ORIENTED_EDGE ( 'NONE', *, *, #51543, .T. ) ;
#67155=FACE_OUTER_BOUND ( 'NONE', #65613, .T. ) ;
#67157=DIRECTION ( 'NONE',  ( 0.000000000000000000, 1.000000000000000000, 0.000000000000000000 ) ) ;
#67257=DIRECTION ( 'NONE',  ( 0.000000000000000000, -0.7071067811865475727, -0.7071067811865475727 ) ) ;
#67271=EDGE_CURVE ( 'NONE', #5944, #43828, #31856, .T. ) ;
#67300=CARTESIAN_POINT ( 'NONE',  ( 76.57571471437145760, 10.00000000000000000, -20.00000000000000000 ) ) ;
#67334=EDGE_CURVE ( 'NONE', #40287, #63181, #40849, .T. ) ;
#67376=VECTOR ( 'NONE', #8373, 1000.000000000000000 ) ;
#67451=LINE ( 'NONE', #57924, #21954 ) ;
#67476=VERTEX_POINT ( 'NONE', #65905 ) ;
#67521=AXIS2_PLACEMENT_3D ( 'NONE', #46528, #39871, #2253 ) ;
#67538=ADVANCED_FACE ( 'NONE', ( #8472 ), #39102, .F. ) ;
#67620=PRODUCT ( 'cutting blade', 'cutting blade', '', ( #10378 ) ) ;
#67716=ORIENTED_EDGE ( 'NONE', *, *, #67334, .F. ) ;
#67730=ORIENTED_EDGE ( 'NONE', *, *, #6986, .T. ) ;
#67745=EDGE_CURVE ( 'NONE', #39369, #23191, #59901, .T. ) ;
#67788=CARTESIAN_POINT ( 'NONE',  ( 76.57571471437145760, 0.000000000000000000, -20.00000000000000000 ) ) ;
#67795=CYLINDRICAL_SURFACE ( 'NONE', #39940, 5.000000000000000888 ) ;
#67807=ORIENTED_EDGE ( 'NONE', *, *, #45276, .T. ) ;
#67960=FACE_OUTER_BOUND ( 'NONE', #39865, .T. ) ;
#68142=VERTEX_POINT ( 'NONE', #30530 ) ;
#68143=ORIENTED_EDGE ( 'NONE', *, *, #8530, .F. ) ;
#68231=DIRECTION ( 'NONE',  ( -0.000000000000000000, -1.000000000000000000, -0.000000000000000000 ) ) ;
#68281=PLANE ( 'NONE',  #4627 ) ;
#68300=EDGE_CURVE ( 'NONE', #23191, #39369, #27365, .T. ) ;
#68568=DIRECTION ( 'NONE',  ( -0.7071067811865475727, -0.7071067811865475727, 3.925231146709437301E-16 ) ) ;
#68607=EDGE_CURVE ( 'NONE', #32425, #44262, #44010, .T. ) ;
#68702=ADVANCED_FACE ( 'NONE', ( #32776 ), #6027, .F. ) ;
#68717=LINE ( 'NONE', #59188, #43820 ) ;
#68723=DIRECTION ( 'NONE',  ( 0.000000000000000000, 0.000000000000000000, -1.000000000000000000 ) ) ;
#68795=FACE_OUTER_BOUND ( 'NONE', #36246, .T. ) ;
#68814=EDGE_CURVE ( 'NONE', #56977, #44262, #28902, .T. ) ;
#68874=CARTESIAN_POINT ( 'NONE',  ( 16.78635691501517613, 6.000000000000000000, -41.68900338898716740 ) ) ;
#68961=DIRECTION ( 'NONE',  ( 0.000000000000000000, 0.000000000000000000, -1.000000000000000000 ) ) ;
#68966=EDGE_LOOP ( 'NONE', ( #65710, #19385, #22686, #38251 ) ) ;
#68985=VECTOR ( 'NONE', #17387, 1000.000000000000000 ) ;
#69002=LINE ( 'NONE', #58121, #5971 ) ;
#69021=DIRECTION ( 'NONE',  ( 0.000000000000000000, 0.000000000000000000, -1.000000000000000000 ) ) ;
#69057=EDGE_CURVE ( 'NONE', #32425, #56977, #26726, .T. ) ;
#69089=VECTOR ( 'NONE', #18794, 1000.000000000000000 ) ;
#69097=EDGE_LOOP ( 'NONE', ( #12754, #28620, #56158, #8625 ) ) ;
#69143=ORIENTED_EDGE ( 'NONE', *, *, #5076, .F. ) ;
#69234=DIRECTION ( 'NONE',  ( -0.000000000000000000, -1.000000000000000000, -0.000000000000000000 ) ) ;
#69245=VECTOR ( 'NONE', #1145, 1000.000000000000114 ) ;
#69248=DIRECTION ( 'NONE',  ( 0.000000000000000000, 0.000000000000000000, -1.000000000000000000 ) ) ;
#69286=EDGE_LOOP ( 'NONE', ( #14048, #55980, #63839 ) ) ;
#69305=ADVANCED_FACE ( 'NONE', ( #20670 ), #56936, .F. ) ;
#69370=VERTEX_POINT ( 'NONE', #20324 ) ;
#69378=DIRECTION ( 'NONE',  ( 0.000000000000000000, 1.000000000000000000, -0.000000000000000000 ) ) ;
#69383=CARTESIAN_POINT ( 'NONE',  ( 50.97490815085634352, 6.000000000000000000, -36.68900338898716740 ) ) ;
#69392=VECTOR ( 'NONE', #23399, 1000.000000000000000 ) ;
#69479=EDGE_LOOP ( 'NONE', ( #35035, #57558, #31065, #26952 ) ) ;
#69481=ADVANCED_FACE ( 'NONE', ( #42468 ), #38578, .F. ) ;
#69536=CARTESIAN_POINT ( 'NONE',  ( 149.0250918491436494, 6.000000000000000000, -41.68900338898718871 ) ) ;
ENDSEC;
END-ISO-10303-21;
